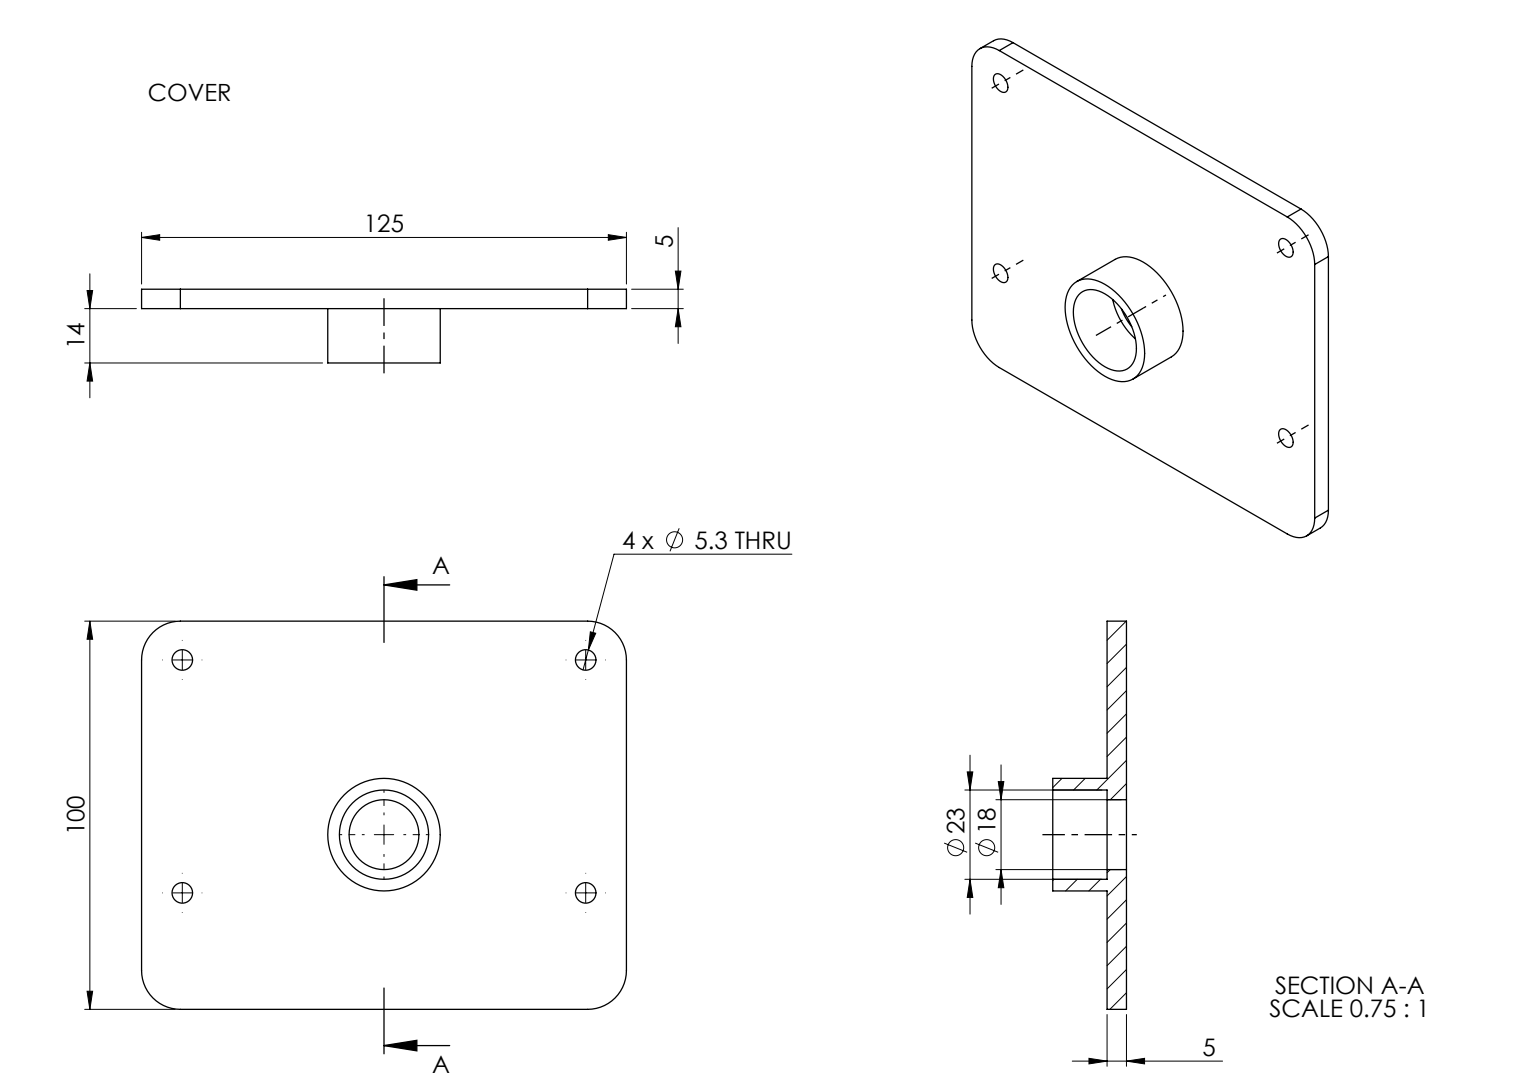
ISO-10303-21;
HEADER;
FILE_DESCRIPTION (('STEP AP214'),
    '1' );
FILE_NAME ('cover.step',
    '2026-10-03T12:29:21',
    ( '' ),
    ( '' ),
    'SwSTEP 2.0',
    'SolidWorks 2026',
    '' );
FILE_SCHEMA (( 'AUTOMOTIVE_DESIGN' ));
ENDSEC;

DATA;
#54=DIRECTION ( 'NONE',  ( 0.000000000000000000, -1.000000000000000000, 0.000000000000000000 ) ) ;
#65=VERTEX_POINT ( 'NONE', #16100 ) ;
#67=CARTESIAN_POINT ( 'NONE',  ( 0.000000000000000000, 0.000000000000000000, 0.000000000000000000 ) ) ;
#103=FILL_AREA_STYLE_COLOUR ( '', #1898 ) ;
#122=CARTESIAN_POINT ( 'NONE',  ( 0.000000000000000000, 0.000000000000000000, 5.000000000000000000 ) ) ;
#132=EDGE_CURVE ( 'NONE', #3302, #4120, #4083, .T. ) ;
#140=FACE_OUTER_BOUND ( 'NONE', #16746, .T. ) ;
#173=DIRECTION ( 'NONE',  ( 0.000000000000000000, 0.000000000000000000, 1.000000000000000000 ) ) ;
#185=DIRECTION ( 'NONE',  ( 1.000000000000000000, 0.000000000000000000, 0.000000000000000000 ) ) ;
#194=DIRECTION ( 'NONE',  ( 1.000000000000000000, 0.000000000000000000, 0.000000000000000000 ) ) ;
#206=( NAMED_UNIT ( * ) SI_UNIT ( $, .STERADIAN. ) SOLID_ANGLE_UNIT ( ) );
#216=LINE ( 'NONE', #11142, #13413 ) ;
#238=CARTESIAN_POINT ( 'NONE',  ( -52.49999999999999289, -30.00000000000000000, 0.000000000000000000 ) ) ;
#249=DIRECTION ( 'NONE',  ( -0.000000000000000000, -0.000000000000000000, 1.000000000000000000 ) ) ;
#257=LINE ( 'NONE', #14576, #12551 ) ;
#270=EDGE_LOOP ( 'NONE', ( #12954, #8026, #4477, #571 ) ) ;
#286=PRODUCT_CONTEXT ( 'NONE', #3554, 'mechanical' ) ;
#314=DIRECTION ( 'NONE',  ( -0.000000000000000000, -0.000000000000000000, 1.000000000000000000 ) ) ;
#324=ORIENTED_EDGE ( 'NONE', *, *, #1202, .T. ) ;
#327=ORIENTED_EDGE ( 'NONE', *, *, #8085, .T. ) ;
#333=DIRECTION ( 'NONE',  ( -1.000000000000000000, 0.000000000000000000, 0.000000000000000000 ) ) ;
#349=VERTEX_POINT ( 'NONE', #17246 ) ;
#368=EDGE_LOOP ( 'NONE', ( #9390, #15256, #3341, #1635, #4917, #19563, #12589, #1221 ) ) ;
#456=DIRECTION ( 'NONE',  ( -0.000000000000000000, -0.000000000000000000, 1.000000000000000000 ) ) ;
#457=AXIS2_PLACEMENT_3D ( 'NONE', #13399, #8610, #18470 ) ;
#459=DIRECTION ( 'NONE',  ( 1.000000000000000000, 0.000000000000000000, 0.000000000000000000 ) ) ;
#487=ORIENTED_EDGE ( 'NONE', *, *, #16093, .F. ) ;
#546=ADVANCED_FACE ( 'NONE', ( #140 ), #19233, .F. ) ;
#571=ORIENTED_EDGE ( 'NONE', *, *, #18719, .T. ) ;
#595=CIRCLE ( 'NONE', #8055, 14.49999999999999822 ) ;
#600=DIRECTION ( 'NONE',  ( 1.000000000000000000, 0.000000000000000000, 0.000000000000000000 ) ) ;
#613=CARTESIAN_POINT ( 'NONE',  ( -54.64999999999999858, -39.99999999999999289, 5.000000000000000000 ) ) ;
#618=DIRECTION ( 'NONE',  ( 0.000000000000000000, 0.000000000000000000, 1.000000000000000000 ) ) ;
#742=VERTEX_POINT ( 'NONE', #7013 ) ;
#768=ORIENTED_EDGE ( 'NONE', *, *, #3979, .F. ) ;
#778=EDGE_CURVE ( 'NONE', #4723, #14352, #12593, .T. ) ;
#848=ORIENTED_EDGE ( 'NONE', *, *, #778, .T. ) ;
#856=FACE_BOUND ( 'NONE', #9647, .T. ) ;
#880=VERTEX_POINT ( 'NONE', #4466 ) ;
#891=MECHANICAL_DESIGN_GEOMETRIC_PRESENTATION_REPRESENTATION('',(#4227),#19831);
#901=ORIENTED_EDGE ( 'NONE', *, *, #12581, .T. ) ;
#929=AXIS2_PLACEMENT_3D ( 'NONE', #67, #17673, #6521 ) ;
#960=DIRECTION ( 'NONE',  ( 0.000000000000000000, 0.000000000000000000, 1.000000000000000000 ) ) ;
#981=SURFACE_STYLE_USAGE ( .BOTH. , #14017 ) ;
#1001=CARTESIAN_POINT ( 'NONE',  ( -62.49999999999999289, -40.00000000000000000, 0.000000000000000000 ) ) ;
#1006=ORIENTED_EDGE ( 'NONE', *, *, #7889, .T. ) ;
#1032=DIRECTION ( 'NONE',  ( 0.000000000000000000, 0.000000000000000000, 1.000000000000000000 ) ) ;
#1035=CARTESIAN_POINT ( 'NONE',  ( 1.040949779275250179E-14, -85.00000000000000000, 19.00000000000000000 ) ) ;
#1057=CARTESIAN_POINT ( 'NONE',  ( 52.00000000000000000, -99.99999999999998579, 5.000000000000000000 ) ) ;
#1061=VERTEX_POINT ( 'NONE', #17520 ) ;
#1065=EDGE_LOOP ( 'NONE', ( #17257, #14549, #3120, #18251 ) ) ;
#1073=ORIENTED_EDGE ( 'NONE', *, *, #4313, .T. ) ;
#1110=CYLINDRICAL_SURFACE ( 'NONE', #14068, 10.00000000000000178 ) ;
#1168=CIRCLE ( 'NONE', #13352, 2.649999999999999467 ) ;
#1190=DIRECTION ( 'NONE',  ( -0.000000000000000000, -0.000000000000000000, 1.000000000000000000 ) ) ;
#1196=FILL_AREA_STYLE ('',( #10623 ) ) ;
#1202=EDGE_CURVE ( 'NONE', #20933, #12828, #18015, .T. ) ;
#1221=ORIENTED_EDGE ( 'NONE', *, *, #7003, .T. ) ;
#1227=VERTEX_POINT ( 'NONE', #3598 ) ;
#1239=DIRECTION ( 'NONE',  ( -0.000000000000000000, 0.000000000000000000, 1.000000000000000000 ) ) ;
#1264=ORIENTED_EDGE ( 'NONE', *, *, #19475, .F. ) ;
#1399=LINE ( 'NONE', #15489, #20347 ) ;
#1407=ORIENTED_EDGE ( 'NONE', *, *, #9613, .T. ) ;
#1414=FACE_BOUND ( 'NONE', #12896, .T. ) ;
#1419=CARTESIAN_POINT ( 'NONE',  ( -52.49999999999999289, -40.00000000000000000, 5.000000000000000000 ) ) ;
#1471=CIRCLE ( 'NONE', #19391, 8.999999999999998224 ) ;
#1510=EDGE_CURVE ( 'NONE', #880, #7974, #1471, .T. ) ;
#1511=LINE ( 'NONE', #14435, #17019 ) ;
#1525=ORIENTED_EDGE ( 'NONE', *, *, #2233, .F. ) ;
#1533=FACE_OUTER_BOUND ( 'NONE', #4714, .T. ) ;
#1548=CARTESIAN_POINT ( 'NONE',  ( 62.49999999999999289, -30.00000000000000000, 5.000000000000000000 ) ) ;
#1551=DIRECTION ( 'NONE',  ( 1.000000000000000000, 0.000000000000000000, 0.000000000000000000 ) ) ;
#1569=FACE_BOUND ( 'NONE', #6597, .T. ) ;
#1633=FACE_OUTER_BOUND ( 'NONE', #20105, .T. ) ;
#1635=ORIENTED_EDGE ( 'NONE', *, *, #6502, .T. ) ;
#1647=CARTESIAN_POINT ( 'NONE',  ( 9.000000000000007105, -85.00000000000000000, 5.000000000000000000 ) ) ;
#1650=ORIENTED_EDGE ( 'NONE', *, *, #1510, .F. ) ;
#1717=VERTEX_POINT ( 'NONE', #20608 ) ;
#1779=ORIENTED_EDGE ( 'NONE', *, *, #5333, .F. ) ;
#1803=SURFACE_STYLE_USAGE ( .BOTH. , #8258 ) ;
#1835=ORIENTED_EDGE ( 'NONE', *, *, #3908, .F. ) ;
#1844=DIRECTION ( 'NONE',  ( 1.000000000000000000, 0.000000000000000000, 0.000000000000000000 ) ) ;
#1855=CARTESIAN_POINT ( 'NONE',  ( 1.040949779275250179E-14, -85.00000000000000000, 5.000000000000000000 ) ) ;
#1898=COLOUR_RGB ( '', 0.66274510, 0.83137255, 0.94901961) ;
#1925=DIRECTION ( 'NONE',  ( -0.000000000000000000, -0.000000000000000000, -1.000000000000000000 ) ) ;
#1974=ADVANCED_FACE ( 'NONE', ( #11586 ), #11485, .F. ) ;
#1980=EDGE_LOOP ( 'NONE', ( #1407, #18308 ) ) ;
#1987=DIRECTION ( 'NONE',  ( 1.000000000000000000, 0.000000000000000000, 0.000000000000000000 ) ) ;
#1998=DIRECTION ( 'NONE',  ( 1.000000000000000000, 0.000000000000000000, -0.000000000000000000 ) ) ;
#2038=DIRECTION ( 'NONE',  ( -0.000000000000000000, 0.000000000000000000, 1.000000000000000000 ) ) ;
#2039=ORIENTED_EDGE ( 'NONE', *, *, #20622, .T. ) ;
#2116=VECTOR ( 'NONE', #12051, 1000.000000000000000 ) ;
#2147=EDGE_CURVE ( 'NONE', #10416, #11011, #18051, .T. ) ;
#2185=CARTESIAN_POINT ( 'NONE',  ( -52.00000000000000000, -39.99999999999999289, 5.000000000000000000 ) ) ;
#2226=EDGE_LOOP ( 'NONE', ( #10599, #3285, #1650, #3524 ) ) ;
#2228=DIRECTION ( 'NONE',  ( -0.000000000000000000, -0.000000000000000000, 1.000000000000000000 ) ) ;
#2229=ORIENTED_EDGE ( 'NONE', *, *, #14858, .F. ) ;
#2233=EDGE_CURVE ( 'NONE', #5012, #8902, #15023, .T. ) ;
#2270=AXIS2_PLACEMENT_3D ( 'NONE', #5785, #4208, #12376 ) ;
#2283=EDGE_LOOP ( 'NONE', ( #8472, #7507, #18183, #15740 ) ) ;
#2337=ORIENTED_EDGE ( 'NONE', *, *, #19059, .T. ) ;
#2376=EDGE_LOOP ( 'NONE', ( #8040, #13146, #1073, #324 ) ) ;
#2402=EDGE_LOOP ( 'NONE', ( #17842, #5849 ) ) ;
#2467=CARTESIAN_POINT ( 'NONE',  ( -11.49999999999998934, -85.00000000000000000, 19.00000000000000000 ) ) ;
#2481=CIRCLE ( 'NONE', #18048, 8.999999999999998224 ) ;
#2500=EDGE_LOOP ( 'NONE', ( #17069, #5268, #8184, #2039 ) ) ;
#2507=DIRECTION ( 'NONE',  ( 1.000000000000000000, 0.000000000000000000, 0.000000000000000000 ) ) ;
#2635=ORIENTED_EDGE ( 'NONE', *, *, #8017, .T. ) ;
#2645=CARTESIAN_POINT ( 'NONE',  ( -52.49999999999999289, -40.00000000000000000, 5.000000000000000000 ) ) ;
#2647=EDGE_CURVE ( 'NONE', #11011, #10416, #20768, .T. ) ;
#2665=ORIENTED_EDGE ( 'NONE', *, *, #5993, .F. ) ;
#2685=ADVANCED_FACE ( 'NONE', ( #16748 ), #5195, .F. ) ;
#2709=CARTESIAN_POINT ( 'NONE',  ( -49.35000000000000142, -99.99999999999998579, 0.000000000000000000 ) ) ;
#2717=CIRCLE ( 'NONE', #4068, 8.999999999999998224 ) ;
#2731=EDGE_CURVE ( 'NONE', #7766, #14029, #20375, .T. ) ;
#2755=ORIENTED_EDGE ( 'NONE', *, *, #6976, .T. ) ;
#2767=AXIS2_PLACEMENT_3D ( 'NONE', #12595, #19062, #7495 ) ;
#2803=ORIENTED_EDGE ( 'NONE', *, *, #8889, .T. ) ;
#2808=EDGE_LOOP ( 'NONE', ( #2337, #15718, #1779, #1264 ) ) ;
#2815=AXIS2_PLACEMENT_3D ( 'NONE', #1548, #5112, #17955 ) ;
#2970=VERTEX_POINT ( 'NONE', #6550 ) ;
#2988=CARTESIAN_POINT ( 'NONE',  ( -54.64999999999999858, -39.99999999999999289, 0.000000000000000000 ) ) ;
#2999=CARTESIAN_POINT ( 'NONE',  ( -62.49999999999999289, -130.0000000000000000, 5.000000000000000000 ) ) ;
#3022=ORIENTED_EDGE ( 'NONE', *, *, #6502, .F. ) ;
#3033=CARTESIAN_POINT ( 'NONE',  ( -62.49999999999999289, -30.00000000000000000, 5.000000000000000000 ) ) ;
#3036=SHAPE_REPRESENTATION ( 'cover', ( #12461 ), #5607 ) ;
#3088=DIRECTION ( 'NONE',  ( -0.000000000000000000, 0.000000000000000000, 1.000000000000000000 ) ) ;
#3120=ORIENTED_EDGE ( 'NONE', *, *, #19475, .T. ) ;
#3173=VECTOR ( 'NONE', #11996, 1000.000000000000000 ) ;
#3218=PLANE ( 'NONE',  #15694 ) ;
#3231=DIRECTION ( 'NONE',  ( 1.000000000000000000, 0.000000000000000000, 0.000000000000000000 ) ) ;
#3285=ORIENTED_EDGE ( 'NONE', *, *, #16985, .T. ) ;
#3293=DIRECTION ( 'NONE',  ( -0.000000000000000000, -0.000000000000000000, 1.000000000000000000 ) ) ;
#3302=VERTEX_POINT ( 'NONE', #11312 ) ;
#3313=AXIS2_PLACEMENT_3D ( 'NONE', #1035, #7484, #9299 ) ;
#3316=VECTOR ( 'NONE', #4614, 1000.000000000000000 ) ;
#3324=DIRECTION ( 'NONE',  ( 1.000000000000000000, 0.000000000000000000, -0.000000000000000000 ) ) ;
#3341=ORIENTED_EDGE ( 'NONE', *, *, #10133, .F. ) ;
#3361=DIRECTION ( 'NONE',  ( 0.000000000000000000, 0.000000000000000000, 1.000000000000000000 ) ) ;
#3401=ORIENTED_EDGE ( 'NONE', *, *, #2147, .T. ) ;
#3461=VECTOR ( 'NONE', #15119, 1000.000000000000000 ) ;
#3476=SHAPE_REPRESENTATION_RELATIONSHIP ( 'NONE' , 'NONE' ,  #3036, #7906 ) ;
#3483=EDGE_CURVE ( 'NONE', #5992, #9439, #11275, .T. ) ;
#3491=DIRECTION ( 'NONE',  ( 1.000000000000000000, 0.000000000000000000, 0.000000000000000000 ) ) ;
#3503=AXIS2_PLACEMENT_3D ( 'NONE', #3622, #456, #6905 ) ;
#3524=ORIENTED_EDGE ( 'NONE', *, *, #13526, .F. ) ;
#3528=CARTESIAN_POINT ( 'NONE',  ( -52.00000000000000000, -99.99999999999998579, 5.000000000000000000 ) ) ;
#3550=PRODUCT_DEFINITION_FORMATION_WITH_SPECIFIED_SOURCE ( 'ANY', '', #18644, .NOT_KNOWN. ) ;
#3554=APPLICATION_CONTEXT ( 'automotive_design' ) ;
#3585=DIRECTION ( 'NONE',  ( 1.000000000000000000, 0.000000000000000000, 0.000000000000000000 ) ) ;
#3594=DIRECTION ( 'NONE',  ( 1.000000000000000000, 0.000000000000000000, 0.000000000000000000 ) ) ;
#3598=CARTESIAN_POINT ( 'NONE',  ( 62.50000000000000000, -120.0000000000000142, 0.000000000000000000 ) ) ;
#3618=CIRCLE ( 'NONE', #11410, 11.50000000000000000 ) ;
#3622=CARTESIAN_POINT ( 'NONE',  ( 52.00000000000000000, -39.99999999999999289, 5.000000000000000000 ) ) ;
#3657=CYLINDRICAL_SURFACE ( 'NONE', #15141, 10.00000000000000178 ) ;
#3684=DIRECTION ( 'NONE',  ( -0.000000000000000000, -0.000000000000000000, -1.000000000000000000 ) ) ;
#3687=( NAMED_UNIT ( * ) PLANE_ANGLE_UNIT ( ) SI_UNIT ( $, .RADIAN. ) );
#3711=CARTESIAN_POINT ( 'NONE',  ( -52.00000000000000000, -99.99999999999998579, 5.000000000000000000 ) ) ;
#3728=LINE ( 'NONE', #4157, #20519 ) ;
#3748=DIRECTION ( 'NONE',  ( -1.000000000000000000, 0.000000000000000000, 0.000000000000000000 ) ) ;
#3874=LINE ( 'NONE', #613, #11834 ) ;
#3878=ORIENTED_EDGE ( 'NONE', *, *, #2731, .F. ) ;
#3880=PLANE ( 'NONE',  #9396 ) ;
#3889=FACE_OUTER_BOUND ( 'NONE', #11532, .T. ) ;
#3908=EDGE_CURVE ( 'NONE', #13107, #2970, #10106, .T. ) ;
#3979=EDGE_CURVE ( 'NONE', #9694, #4085, #257, .T. ) ;
#4002=DIRECTION ( 'NONE',  ( 1.000000000000000000, 0.000000000000000000, 0.000000000000000000 ) ) ;
#4016=FACE_BOUND ( 'NONE', #2402, .T. ) ;
#4023=PRODUCT_DEFINITION ( 'UNKNOWN', '', #3550, #5590 ) ;
#4051=CYLINDRICAL_SURFACE ( 'NONE', #16717, 14.49999999999999822 ) ;
#4068=AXIS2_PLACEMENT_3D ( 'NONE', #18351, #11993, #5102 ) ;
#4083=LINE ( 'NONE', #7161, #2116 ) ;
#4085=VERTEX_POINT ( 'NONE', #18364 ) ;
#4110=CYLINDRICAL_SURFACE ( 'NONE', #18878, 2.649999999999999467 ) ;
#4120=VERTEX_POINT ( 'NONE', #10204 ) ;
#4157=CARTESIAN_POINT ( 'NONE',  ( -8.999999999999987566, -85.00000000000000000, 5.000000000000000000 ) ) ;
#4208=DIRECTION ( 'NONE',  ( -0.000000000000000000, 0.000000000000000000, 1.000000000000000000 ) ) ;
#4227=STYLED_ITEM ( 'NONE', ( #5072 ), #7906 ) ;
#4257=AXIS2_PLACEMENT_3D ( 'NONE', #14702, #173, #16386 ) ;
#4273=DIRECTION ( 'NONE',  ( 0.000000000000000000, 0.000000000000000000, -1.000000000000000000 ) ) ;
#4277=FACE_OUTER_BOUND ( 'NONE', #7762, .T. ) ;
#4298=ADVANCED_FACE ( 'NONE', ( #1414, #1633 ), #16236, .T. ) ;
#4313=EDGE_CURVE ( 'NONE', #18213, #20933, #16332, .T. ) ;
#4338=DIRECTION ( 'NONE',  ( -0.000000000000000000, -0.000000000000000000, 1.000000000000000000 ) ) ;
#4344=ORIENTED_EDGE ( 'NONE', *, *, #132, .F. ) ;
#4405=ORIENTED_EDGE ( 'NONE', *, *, #13384, .T. ) ;
#4452=CARTESIAN_POINT ( 'NONE',  ( 49.35000000000000142, -39.99999999999999289, 5.000000000000000000 ) ) ;
#4466=CARTESIAN_POINT ( 'NONE',  ( -8.999999999999987566, -85.00000000000000000, 0.000000000000000000 ) ) ;
#4477=ORIENTED_EDGE ( 'NONE', *, *, #8889, .F. ) ;
#4501=DIRECTION ( 'NONE',  ( -0.000000000000000000, -0.000000000000000000, 1.000000000000000000 ) ) ;
#4545=DIRECTION ( 'NONE',  ( 1.000000000000000000, 0.000000000000000000, 0.000000000000000000 ) ) ;
#4576=DIRECTION ( 'NONE',  ( -0.000000000000000000, -0.000000000000000000, 1.000000000000000000 ) ) ;
#4585=CARTESIAN_POINT ( 'NONE',  ( -52.00000000000000000, -99.99999999999998579, 0.000000000000000000 ) ) ;
#4613=VECTOR ( 'NONE', #1190, 1000.000000000000000 ) ;
#4614=DIRECTION ( 'NONE',  ( -0.000000000000000000, -0.000000000000000000, 1.000000000000000000 ) ) ;
#4660=DIRECTION ( 'NONE',  ( 1.000000000000000000, 0.000000000000000000, 0.000000000000000000 ) ) ;
#4714=EDGE_LOOP ( 'NONE', ( #14546, #16819, #2635, #17037 ) ) ;
#4723=VERTEX_POINT ( 'NONE', #15893 ) ;
#4730=DIRECTION ( 'NONE',  ( 0.000000000000000000, 0.000000000000000000, 1.000000000000000000 ) ) ;
#4732=CIRCLE ( 'NONE', #16246, 14.49999999999999822 ) ;
#4757=VERTEX_POINT ( 'NONE', #16305 ) ;
#4781=CARTESIAN_POINT ( 'NONE',  ( 49.35000000000000142, -99.99999999999998579, 5.000000000000000000 ) ) ;
#4810=CIRCLE ( 'NONE', #2767, 2.649999999999999467 ) ;
#4838=FACE_OUTER_BOUND ( 'NONE', #368, .T. ) ;
#4897=DIRECTION ( 'NONE',  ( -0.000000000000000000, -0.000000000000000000, 1.000000000000000000 ) ) ;
#4901=DIRECTION ( 'NONE',  ( -0.000000000000000000, -0.000000000000000000, -1.000000000000000000 ) ) ;
#4917=ORIENTED_EDGE ( 'NONE', *, *, #9430, .F. ) ;
#5012=VERTEX_POINT ( 'NONE', #18627 ) ;
#5027=ORIENTED_EDGE ( 'NONE', *, *, #132, .T. ) ;
#5040=ORIENTED_EDGE ( 'NONE', *, *, #12921, .T. ) ;
#5072=PRESENTATION_STYLE_ASSIGNMENT (( #1803 ) ) ;
#5102=DIRECTION ( 'NONE',  ( 1.000000000000000000, 0.000000000000000000, 0.000000000000000000 ) ) ;
#5104=DIRECTION ( 'NONE',  ( -1.000000000000000000, -0.000000000000000000, -0.000000000000000000 ) ) ;
#5112=DIRECTION ( 'NONE',  ( -1.000000000000000000, -6.938893903907228378E-17, 0.000000000000000000 ) ) ;
#5113=EDGE_LOOP ( 'NONE', ( #5452, #8295, #1006, #18242 ) ) ;
#5174=DIRECTION ( 'NONE',  ( 0.000000000000000000, 0.000000000000000000, 1.000000000000000000 ) ) ;
#5175=CARTESIAN_POINT ( 'NONE',  ( 52.00000000000000000, -39.99999999999999289, 5.000000000000000000 ) ) ;
#5195=CYLINDRICAL_SURFACE ( 'NONE', #17686, 2.649999999999999467 ) ;
#5217=CARTESIAN_POINT ( 'NONE',  ( -49.35000000000000142, -99.99999999999998579, 5.000000000000000000 ) ) ;
#5267=AXIS2_PLACEMENT_3D ( 'NONE', #15050, #13251, #3594 ) ;
#5268=ORIENTED_EDGE ( 'NONE', *, *, #14560, .F. ) ;
#5293=CIRCLE ( 'NONE', #14825, 11.50000000000000000 ) ;
#5303=PLANE ( 'NONE',  #9025 ) ;
#5329=DIRECTION ( 'NONE',  ( 0.000000000000000000, -0.000000000000000000, 1.000000000000000000 ) ) ;
#5333=EDGE_CURVE ( 'NONE', #19867, #12993, #17798, .T. ) ;
#5340=EDGE_LOOP ( 'NONE', ( #9730, #6806 ) ) ;
#5425=DIRECTION ( 'NONE',  ( -0.000000000000000000, -0.000000000000000000, -1.000000000000000000 ) ) ;
#5432=VECTOR ( 'NONE', #5329, 1000.000000000000000 ) ;
#5446=CARTESIAN_POINT ( 'NONE',  ( 9.000000000000007105, -85.00000000000000000, 0.000000000000000000 ) ) ;
#5452=ORIENTED_EDGE ( 'NONE', *, *, #2647, .F. ) ;
#5538=DIRECTION ( 'NONE',  ( 1.000000000000000000, 0.000000000000000000, 0.000000000000000000 ) ) ;
#5584=CARTESIAN_POINT ( 'NONE',  ( 1.040949779275250179E-14, -85.00000000000000000, 5.000000000000000000 ) ) ;
#5590=PRODUCT_DEFINITION_CONTEXT ( 'detailed design', #18739, 'design' ) ;
#5606=CARTESIAN_POINT ( 'NONE',  ( -52.00000000000000000, -39.99999999999999289, 0.000000000000000000 ) ) ;
#5607=( GEOMETRIC_REPRESENTATION_CONTEXT ( 3 ) GLOBAL_UNCERTAINTY_ASSIGNED_CONTEXT ( ( #13245 ) ) GLOBAL_UNIT_ASSIGNED_CONTEXT ( ( #16006, #17399, #206 ) ) REPRESENTATION_CONTEXT ( 'NONE', 'WORKASPACE' ) );
#5642=ORIENTED_EDGE ( 'NONE', *, *, #12153, .F. ) ;
#5672=CARTESIAN_POINT ( 'NONE',  ( -62.49999999999999289, -40.00000000000000000, 5.000000000000000000 ) ) ;
#5701=DIRECTION ( 'NONE',  ( -0.000000000000000000, -0.000000000000000000, 1.000000000000000000 ) ) ;
#5710=ADVANCED_FACE ( 'NONE', ( #6894 ), #19721, .T. ) ;
#5768=VECTOR ( 'NONE', #4897, 1000.000000000000000 ) ;
#5770=EDGE_CURVE ( 'NONE', #65, #12993, #11564, .T. ) ;
#5785=CARTESIAN_POINT ( 'NONE',  ( 52.00000000000000000, -99.99999999999998579, 0.000000000000000000 ) ) ;
#5813=AXIS2_PLACEMENT_3D ( 'NONE', #15275, #2038, #459 ) ;
#5837=( LENGTH_UNIT ( ) NAMED_UNIT ( * ) SI_UNIT ( .MILLI., .METRE. ) );
#5849=ORIENTED_EDGE ( 'NONE', *, *, #17993, .F. ) ;
#5880=CARTESIAN_POINT ( 'NONE',  ( -14.49999999999998934, -85.00000000000000000, 19.00000000000000000 ) ) ;
#5899=DIRECTION ( 'NONE',  ( -0.000000000000000000, -0.000000000000000000, 1.000000000000000000 ) ) ;
#5957=CIRCLE ( 'NONE', #8653, 14.49999999999999822 ) ;
#5992=VERTEX_POINT ( 'NONE', #20461 ) ;
#5993=EDGE_CURVE ( 'NONE', #4723, #16392, #18982, .T. ) ;
#6071=ORIENTED_EDGE ( 'NONE', *, *, #2647, .T. ) ;
#6085=ORIENTED_EDGE ( 'NONE', *, *, #13384, .F. ) ;
#6109=ORIENTED_EDGE ( 'NONE', *, *, #7606, .F. ) ;
#6133=CYLINDRICAL_SURFACE ( 'NONE', #10043, 11.50000000000000000 ) ;
#6190=LINE ( 'NONE', #5880, #18085 ) ;
#6230=AXIS2_PLACEMENT_3D ( 'NONE', #3711, #13383, #15268 ) ;
#6300=CYLINDRICAL_SURFACE ( 'NONE', #7849, 10.00000000000000178 ) ;
#6308=ADVANCED_FACE ( 'NONE', ( #3889 ), #10370, .F. ) ;
#6329=CIRCLE ( 'NONE', #9721, 11.50000000000000000 ) ;
#6385=DIRECTION ( 'NONE',  ( -0.000000000000000000, -0.000000000000000000, 1.000000000000000000 ) ) ;
#6438=DIRECTION ( 'NONE',  ( 0.000000000000000000, 0.000000000000000000, 1.000000000000000000 ) ) ;
#6470=EDGE_LOOP ( 'NONE', ( #10872, #11075, #10292, #10874 ) ) ;
#6494=VECTOR ( 'NONE', #7893, 1000.000000000000000 ) ;
#6496=AXIS2_PLACEMENT_3D ( 'NONE', #13472, #6880, #18022 ) ;
#6502=EDGE_CURVE ( 'NONE', #1227, #15433, #17175, .T. ) ;
#6521=DIRECTION ( 'NONE',  ( 1.000000000000000000, 0.000000000000000000, 0.000000000000000000 ) ) ;
#6550=CARTESIAN_POINT ( 'NONE',  ( -62.49999999999999289, -120.0000000000000142, 5.000000000000000000 ) ) ;
#6555=ORIENTED_EDGE ( 'NONE', *, *, #10108, .T. ) ;
#6560=( NAMED_UNIT ( * ) SI_UNIT ( $, .STERADIAN. ) SOLID_ANGLE_UNIT ( ) );
#6562=DIRECTION ( 'NONE',  ( -6.938893903907228378E-17, 1.000000000000000000, -0.000000000000000000 ) ) ;
#6574=LINE ( 'NONE', #4781, #8598 ) ;
#6588=DIRECTION ( 'NONE',  ( -0.000000000000000000, -0.000000000000000000, -1.000000000000000000 ) ) ;
#6591=CARTESIAN_POINT ( 'NONE',  ( 1.040949779275250179E-14, -85.00000000000000000, 19.00000000000000000 ) ) ;
#6597=EDGE_LOOP ( 'NONE', ( #7651, #14778 ) ) ;
#6602=DIRECTION ( 'NONE',  ( -0.000000000000000000, -0.000000000000000000, 1.000000000000000000 ) ) ;
#6735=FACE_OUTER_BOUND ( 'NONE', #6470, .T. ) ;
#6794=DIRECTION ( 'NONE',  ( 1.000000000000000000, 0.000000000000000000, 0.000000000000000000 ) ) ;
#6806=ORIENTED_EDGE ( 'NONE', *, *, #11279, .T. ) ;
#6818=CIRCLE ( 'NONE', #16984, 10.00000000000000178 ) ;
#6880=DIRECTION ( 'NONE',  ( -0.000000000000000000, -0.000000000000000000, 1.000000000000000000 ) ) ;
#6890=FACE_BOUND ( 'NONE', #9412, .T. ) ;
#6894=FACE_OUTER_BOUND ( 'NONE', #15648, .T. ) ;
#6905=DIRECTION ( 'NONE',  ( 1.000000000000000000, 0.000000000000000000, 0.000000000000000000 ) ) ;
#6933=EDGE_LOOP ( 'NONE', ( #12931, #1835, #10041, #11228 ) ) ;
#6976=EDGE_CURVE ( 'NONE', #14029, #4120, #10974, .T. ) ;
#7003=EDGE_CURVE ( 'NONE', #10860, #9694, #19884, .T. ) ;
#7013=CARTESIAN_POINT ( 'NONE',  ( -14.49999999999998934, -85.00000000000000000, 5.000000000000000000 ) ) ;
#7072=DIRECTION ( 'NONE',  ( 0.000000000000000000, -0.000000000000000000, -1.000000000000000000 ) ) ;
#7161=CARTESIAN_POINT ( 'NONE',  ( 62.49999999999999289, -30.00000000000000000, 5.000000000000000000 ) ) ;
#7194=DIRECTION ( 'NONE',  ( -0.000000000000000000, 0.000000000000000000, 1.000000000000000000 ) ) ;
#7246=CARTESIAN_POINT ( 'NONE',  ( 14.50000000000000888, -85.00000000000000000, 19.00000000000000000 ) ) ;
#7309=FACE_OUTER_BOUND ( 'NONE', #10689, .T. ) ;
#7311=ORIENTED_EDGE ( 'NONE', *, *, #11837, .T. ) ;
#7326=ORIENTED_EDGE ( 'NONE', *, *, #3483, .T. ) ;
#7404=CARTESIAN_POINT ( 'NONE',  ( -52.49999999999999289, -120.0000000000000142, 0.000000000000000000 ) ) ;
#7445=DIRECTION ( 'NONE',  ( -0.000000000000000000, -0.000000000000000000, 1.000000000000000000 ) ) ;
#7449=ORIENTED_EDGE ( 'NONE', *, *, #778, .F. ) ;
#7484=DIRECTION ( 'NONE',  ( -0.000000000000000000, -0.000000000000000000, -1.000000000000000000 ) ) ;
#7495=DIRECTION ( 'NONE',  ( 1.000000000000000000, 0.000000000000000000, 0.000000000000000000 ) ) ;
#7507=ORIENTED_EDGE ( 'NONE', *, *, #12601, .T. ) ;
#7538=ORIENTED_EDGE ( 'NONE', *, *, #20247, .F. ) ;
#7548=PLANE ( 'NONE',  #13124 ) ;
#7574=AXIS2_PLACEMENT_3D ( 'NONE', #17587, #4338, #4545 ) ;
#7606=EDGE_CURVE ( 'NONE', #65, #13495, #5293, .T. ) ;
#7646=ORIENTED_EDGE ( 'NONE', *, *, #1510, .T. ) ;
#7651=ORIENTED_EDGE ( 'NONE', *, *, #12153, .T. ) ;
#7684=DIRECTION ( 'NONE',  ( -0.000000000000000000, -0.000000000000000000, -1.000000000000000000 ) ) ;
#7762=EDGE_LOOP ( 'NONE', ( #2665, #16982, #14718, #6555 ) ) ;
#7766=VERTEX_POINT ( 'NONE', #13552 ) ;
#7849=AXIS2_PLACEMENT_3D ( 'NONE', #12790, #8002, #14482 ) ;
#7871=EDGE_CURVE ( 'NONE', #4085, #4757, #6818, .T. ) ;
#7873=DIRECTION ( 'NONE',  ( 0.000000000000000000, 0.000000000000000000, -1.000000000000000000 ) ) ;
#7875=CARTESIAN_POINT ( 'NONE',  ( 52.00000000000000000, -39.99999999999999289, 5.000000000000000000 ) ) ;
#7884=ORIENTED_EDGE ( 'NONE', *, *, #18932, .T. ) ;
#7889=EDGE_CURVE ( 'NONE', #10195, #18098, #4810, .T. ) ;
#7892=ORIENTED_EDGE ( 'NONE', *, *, #11204, .F. ) ;
#7893=DIRECTION ( 'NONE',  ( -1.000000000000000000, -0.000000000000000000, -0.000000000000000000 ) ) ;
#7906=ADVANCED_BREP_SHAPE_REPRESENTATION ( '', ( #17220, #12461 ), #5607 ) ;
#7914=CIRCLE ( 'NONE', #14695, 2.649999999999999467 ) ;
#7918=DIRECTION ( 'NONE',  ( 1.000000000000000000, 0.000000000000000000, 0.000000000000000000 ) ) ;
#7949=AXIS2_PLACEMENT_3D ( 'NONE', #13257, #3088, #3491 ) ;
#7974=VERTEX_POINT ( 'NONE', #5446 ) ;
#7983=PLANE ( 'NONE',  #16662 ) ;
#7992=DIRECTION ( 'NONE',  ( 0.000000000000000000, 0.000000000000000000, 1.000000000000000000 ) ) ;
#8002=DIRECTION ( 'NONE',  ( -0.000000000000000000, 0.000000000000000000, -1.000000000000000000 ) ) ;
#8017=EDGE_CURVE ( 'NONE', #7766, #9694, #20400, .T. ) ;
#8022=CIRCLE ( 'NONE', #2270, 2.649999999999999467 ) ;
#8026=ORIENTED_EDGE ( 'NONE', *, *, #12068, .T. ) ;
#8040=ORIENTED_EDGE ( 'NONE', *, *, #12601, .F. ) ;
#8041=AXIS2_PLACEMENT_3D ( 'NONE', #8892, #16628, #15153 ) ;
#8055=AXIS2_PLACEMENT_3D ( 'NONE', #17271, #960, #4002 ) ;
#8067=DIRECTION ( 'NONE',  ( 1.000000000000000000, 0.000000000000000000, 0.000000000000000000 ) ) ;
#8079=DIRECTION ( 'NONE',  ( -0.000000000000000000, -0.000000000000000000, 1.000000000000000000 ) ) ;
#8085=EDGE_CURVE ( 'NONE', #14352, #4723, #20703, .T. ) ;
#8089=ADVANCED_FACE ( 'NONE', ( #20819 ), #6300, .T. ) ;
#8140=CARTESIAN_POINT ( 'NONE',  ( -11.49999999999998934, -85.00000000000000000, 5.000000000000000000 ) ) ;
#8163=AXIS2_PLACEMENT_3D ( 'NONE', #14475, #249, #9787 ) ;
#8184=ORIENTED_EDGE ( 'NONE', *, *, #11919, .T. ) ;
#8203=ADVANCED_FACE ( 'NONE', ( #1533 ), #7983, .F. ) ;
#8258=SURFACE_SIDE_STYLE ('',( #16415 ) ) ;
#8260=CYLINDRICAL_SURFACE ( 'NONE', #12236, 2.649999999999999467 ) ;
#8263=ADVANCED_FACE ( 'NONE', ( #20906 ), #13242, .F. ) ;
#8295=ORIENTED_EDGE ( 'NONE', *, *, #17680, .T. ) ;
#8325=DIRECTION ( 'NONE',  ( -0.000000000000000000, -0.000000000000000000, 1.000000000000000000 ) ) ;
#8364=( LENGTH_UNIT ( ) NAMED_UNIT ( * ) SI_UNIT ( .MILLI., .METRE. ) );
#8384=EDGE_LOOP ( 'NONE', ( #7892, #17588, #3878, #16103 ) ) ;
#8465=VERTEX_POINT ( 'NONE', #9103 ) ;
#8471=DIRECTION ( 'NONE',  ( 0.000000000000000000, -0.000000000000000000, -1.000000000000000000 ) ) ;
#8472=ORIENTED_EDGE ( 'NONE', *, *, #20095, .F. ) ;
#8493=DIRECTION ( 'NONE',  ( -0.000000000000000000, 0.000000000000000000, 1.000000000000000000 ) ) ;
#8533=DIRECTION ( 'NONE',  ( 1.000000000000000000, 0.000000000000000000, 0.000000000000000000 ) ) ;
#8568=UNCERTAINTY_MEASURE_WITH_UNIT (LENGTH_MEASURE( 1.000000000000000082E-05 ), #8364, 'distance_accuracy_value', 'NONE');
#8598=VECTOR ( 'NONE', #8079, 1000.000000000000000 ) ;
#8610=DIRECTION ( 'NONE',  ( -0.000000000000000000, 0.000000000000000000, 1.000000000000000000 ) ) ;
#8653=AXIS2_PLACEMENT_3D ( 'NONE', #18841, #1032, #17247 ) ;
#8696=ADVANCED_FACE ( 'NONE', ( #6735 ), #11510, .F. ) ;
#8864=FACE_OUTER_BOUND ( 'NONE', #5340, .T. ) ;
#8889=EDGE_CURVE ( 'NONE', #8465, #11004, #8964, .T. ) ;
#8892=CARTESIAN_POINT ( 'NONE',  ( -52.49999999999999289, -120.0000000000000142, 5.000000000000000000 ) ) ;
#8902=VERTEX_POINT ( 'NONE', #2709 ) ;
#8925=EDGE_CURVE ( 'NONE', #4757, #10860, #10673, .T. ) ;
#8941=LINE ( 'NONE', #18695, #10285 ) ;
#8964=LINE ( 'NONE', #17236, #10592 ) ;
#9003=CIRCLE ( 'NONE', #5267, 10.00000000000000178 ) ;
#9019=EDGE_LOOP ( 'NONE', ( #9158, #2755, #4344, #19574 ) ) ;
#9025=AXIS2_PLACEMENT_3D ( 'NONE', #13793, #20243, #18240 ) ;
#9053=CARTESIAN_POINT ( 'NONE',  ( 1.040949779275250179E-14, -85.00000000000000000, 19.00000000000000000 ) ) ;
#9073=ORIENTED_EDGE ( 'NONE', *, *, #20247, .T. ) ;
#9103=CARTESIAN_POINT ( 'NONE',  ( -52.49999999999999289, -130.0000000000000000, 5.000000000000000000 ) ) ;
#9112=DIRECTION ( 'NONE',  ( 0.000000000000000000, -0.000000000000000000, -1.000000000000000000 ) ) ;
#9158=ORIENTED_EDGE ( 'NONE', *, *, #10133, .T. ) ;
#9163=EDGE_CURVE ( 'NONE', #9439, #5992, #2481, .T. ) ;
#9190=COLOUR_RGB ( '', 0.66274510, 0.83137255, 0.94901961) ;
#9212=CARTESIAN_POINT ( 'NONE',  ( 1.040949779275250179E-14, -85.00000000000000000, 19.00000000000000000 ) ) ;
#9260=LINE ( 'NONE', #20688, #14383 ) ;
#9262=CYLINDRICAL_SURFACE ( 'NONE', #17408, 2.649999999999999467 ) ;
#9299=DIRECTION ( 'NONE',  ( -1.000000000000000000, 0.000000000000000000, 0.000000000000000000 ) ) ;
#9305=CARTESIAN_POINT ( 'NONE',  ( 52.50000000000000000, -120.0000000000000142, 0.000000000000000000 ) ) ;
#9390=ORIENTED_EDGE ( 'NONE', *, *, #8017, .F. ) ;
#9392=CIRCLE ( 'NONE', #8041, 10.00000000000000178 ) ;
#9396=AXIS2_PLACEMENT_3D ( 'NONE', #10360, #618, #1998 ) ;
#9400=AXIS2_PLACEMENT_3D ( 'NONE', #20822, #17960, #11392 ) ;
#9412=EDGE_LOOP ( 'NONE', ( #11224, #2229 ) ) ;
#9430=EDGE_CURVE ( 'NONE', #19301, #15433, #8941, .T. ) ;
#9439=VERTEX_POINT ( 'NONE', #15407 ) ;
#9458=DIRECTION ( 'NONE',  ( 0.000000000000000000, 1.000000000000000000, 0.000000000000000000 ) ) ;
#9468=ORIENTED_EDGE ( 'NONE', *, *, #3483, .F. ) ;
#9483=CARTESIAN_POINT ( 'NONE',  ( 52.00000000000000000, -39.99999999999999289, 0.000000000000000000 ) ) ;
#9486=ADVANCED_FACE ( 'NONE', ( #4277 ), #9262, .F. ) ;
#9566=DIRECTION ( 'NONE',  ( 0.000000000000000000, 0.000000000000000000, -1.000000000000000000 ) ) ;
#9613=EDGE_CURVE ( 'NONE', #18213, #349, #7914, .T. ) ;
#9634=DIRECTION ( 'NONE',  ( -0.000000000000000000, -0.000000000000000000, 1.000000000000000000 ) ) ;
#9647=EDGE_LOOP ( 'NONE', ( #6085, #16166 ) ) ;
#9662=DIRECTION ( 'NONE',  ( -0.000000000000000000, 0.000000000000000000, -1.000000000000000000 ) ) ;
#9694=VERTEX_POINT ( 'NONE', #238 ) ;
#9695=CARTESIAN_POINT ( 'NONE',  ( -62.49999999999999289, -120.0000000000000142, 5.000000000000000000 ) ) ;
#9721=AXIS2_PLACEMENT_3D ( 'NONE', #15994, #16299, #194 ) ;
#9730=ORIENTED_EDGE ( 'NONE', *, *, #14560, .T. ) ;
#9761=LINE ( 'NONE', #18018, #14398 ) ;
#9787=DIRECTION ( 'NONE',  ( 1.000000000000000000, 0.000000000000000000, 0.000000000000000000 ) ) ;
#9839=ORIENTED_EDGE ( 'NONE', *, *, #17993, .T. ) ;
#9845=FILL_AREA_STYLE ('',( #103 ) ) ;
#9875=EDGE_CURVE ( 'NONE', #1717, #18188, #19766, .T. ) ;
#9890=ORIENTED_EDGE ( 'NONE', *, *, #14826, .T. ) ;
#9953=CARTESIAN_POINT ( 'NONE',  ( -52.00000000000000000, -39.99999999999999289, 5.000000000000000000 ) ) ;
#9955=AXIS2_PLACEMENT_3D ( 'NONE', #19950, #7445, #13926 ) ;
#9969=VERTEX_POINT ( 'NONE', #20464 ) ;
#9984=EDGE_CURVE ( 'NONE', #3302, #1227, #1399, .T. ) ;
#10041=ORIENTED_EDGE ( 'NONE', *, *, #19081, .F. ) ;
#10043=AXIS2_PLACEMENT_3D ( 'NONE', #12292, #12615, #18767 ) ;
#10060=VECTOR ( 'NONE', #8325, 1000.000000000000000 ) ;
#10062=DIRECTION ( 'NONE',  ( 1.000000000000000000, 0.000000000000000000, 0.000000000000000000 ) ) ;
#10106=LINE ( 'NONE', #9695, #5432 ) ;
#10108=EDGE_CURVE ( 'NONE', #1061, #16392, #10546, .T. ) ;
#10113=ADVANCED_FACE ( 'NONE', ( #11350 ), #11541, .F. ) ;
#10133=EDGE_CURVE ( 'NONE', #1227, #14029, #1511, .T. ) ;
#10141=ADVANCED_FACE ( 'NONE', ( #17822 ), #8260, .F. ) ;
#10159=VECTOR ( 'NONE', #6588, 1000.000000000000000 ) ;
#10161=DIRECTION ( 'NONE',  ( 0.000000000000000000, -1.000000000000000000, 0.000000000000000000 ) ) ;
#10195=VERTEX_POINT ( 'NONE', #12074 ) ;
#10204=CARTESIAN_POINT ( 'NONE',  ( 62.49999999999999289, -40.00000000000000000, 5.000000000000000000 ) ) ;
#10275=EDGE_CURVE ( 'NONE', #4757, #2970, #18322, .T. ) ;
#10285=VECTOR ( 'NONE', #5538, 1000.000000000000000 ) ;
#10292=ORIENTED_EDGE ( 'NONE', *, *, #14776, .T. ) ;
#10360=CARTESIAN_POINT ( 'NONE',  ( 1.040949779275250179E-14, -85.00000000000000000, 19.00000000000000000 ) ) ;
#10370=CYLINDRICAL_SURFACE ( 'NONE', #17848, 8.999999999999998224 ) ;
#10416=VERTEX_POINT ( 'NONE', #16480 ) ;
#10421=CIRCLE ( 'NONE', #12451, 2.649999999999999467 ) ;
#10429=ORIENTED_EDGE ( 'NONE', *, *, #5993, .T. ) ;
#10444=ORIENTED_EDGE ( 'NONE', *, *, #8925, .T. ) ;
#10481=UNCERTAINTY_MEASURE_WITH_UNIT (LENGTH_MEASURE( 1.000000000000000082E-05 ), #5837, 'distance_accuracy_value', 'NONE');
#10497=FACE_BOUND ( 'NONE', #14926, .T. ) ;
#10546=CIRCLE ( 'NONE', #14946, 2.649999999999999467 ) ;
#10554=( GEOMETRIC_REPRESENTATION_CONTEXT ( 3 ) GLOBAL_UNCERTAINTY_ASSIGNED_CONTEXT ( ( #10481 ) ) GLOBAL_UNIT_ASSIGNED_CONTEXT ( ( #5837, #10732, #17197 ) ) REPRESENTATION_CONTEXT ( 'NONE', 'WORKASPACE' ) );
#10576=EDGE_LOOP ( 'NONE', ( #20411, #20444, #3022, #11146 ) ) ;
#10592=VECTOR ( 'NONE', #2507, 1000.000000000000000 ) ;
#10599=ORIENTED_EDGE ( 'NONE', *, *, #9163, .T. ) ;
#10623=FILL_AREA_STYLE_COLOUR ( '', #9190 ) ;
#10673=LINE ( 'NONE', #5672, #3461 ) ;
#10689=EDGE_LOOP ( 'NONE', ( #5027, #15214, #11790, #16228, #16214, #7884, #2803, #901 ) ) ;
#10732=( NAMED_UNIT ( * ) PLANE_ANGLE_UNIT ( ) SI_UNIT ( $, .RADIAN. ) );
#10774=ADVANCED_FACE ( 'NONE', ( #20798 ), #1110, .T. ) ;
#10788=ADVANCED_FACE ( 'NONE', ( #14039 ), #14241, .T. ) ;
#10860=VERTEX_POINT ( 'NONE', #1001 ) ;
#10872=ORIENTED_EDGE ( 'NONE', *, *, #17680, .F. ) ;
#10874=ORIENTED_EDGE ( 'NONE', *, *, #16093, .T. ) ;
#10921=EDGE_CURVE ( 'NONE', #14352, #1061, #15700, .T. ) ;
#10941=DIRECTION ( 'NONE',  ( 1.000000000000000000, 0.000000000000000000, 0.000000000000000000 ) ) ;
#10953=DIRECTION ( 'NONE',  ( 1.000000000000000000, 0.000000000000000000, 0.000000000000000000 ) ) ;
#10961=DIRECTION ( 'NONE',  ( 0.000000000000000000, 0.000000000000000000, 1.000000000000000000 ) ) ;
#10974=LINE ( 'NONE', #17016, #3316 ) ;
#11004=VERTEX_POINT ( 'NONE', #11037 ) ;
#11011=VERTEX_POINT ( 'NONE', #2988 ) ;
#11037=CARTESIAN_POINT ( 'NONE',  ( 52.50000000000000000, -130.0000000000000000, 5.000000000000000000 ) ) ;
#11059=CARTESIAN_POINT ( 'NONE',  ( 52.50000000000000000, -120.0000000000000142, 5.000000000000000000 ) ) ;
#11075=ORIENTED_EDGE ( 'NONE', *, *, #2147, .F. ) ;
#11092=ORIENTED_EDGE ( 'NONE', *, *, #11279, .F. ) ;
#11142=CARTESIAN_POINT ( 'NONE',  ( -62.49999999999999289, -30.00000000000000000, 0.000000000000000000 ) ) ;
#11146=ORIENTED_EDGE ( 'NONE', *, *, #9984, .F. ) ;
#11168=EDGE_CURVE ( 'NONE', #10860, #13107, #216, .T. ) ;
#11188=EDGE_LOOP ( 'NONE', ( #7449, #10429, #9890, #15166 ) ) ;
#11199=FACE_BOUND ( 'NONE', #1980, .T. ) ;
#11204=EDGE_CURVE ( 'NONE', #4120, #18964, #9003, .T. ) ;
#11224=ORIENTED_EDGE ( 'NONE', *, *, #1202, .F. ) ;
#11228=ORIENTED_EDGE ( 'NONE', *, *, #18719, .F. ) ;
#11236=CARTESIAN_POINT ( 'NONE',  ( 52.00000000000000000, -39.99999999999999289, 5.000000000000000000 ) ) ;
#11275=CIRCLE ( 'NONE', #16013, 8.999999999999998224 ) ;
#11279=EDGE_CURVE ( 'NONE', #9969, #16951, #5957, .T. ) ;
#11312=CARTESIAN_POINT ( 'NONE',  ( 62.50000000000000000, -120.0000000000000142, 5.000000000000000000 ) ) ;
#11322=VECTOR ( 'NONE', #5104, 1000.000000000000000 ) ;
#11350=FACE_OUTER_BOUND ( 'NONE', #2226, .T. ) ;
#11392=DIRECTION ( 'NONE',  ( 1.000000000000000000, 0.000000000000000000, 0.000000000000000000 ) ) ;
#11410=AXIS2_PLACEMENT_3D ( 'NONE', #9212, #4730, #19350 ) ;
#11485=PLANE ( 'NONE',  #2815 ) ;
#11510=CYLINDRICAL_SURFACE ( 'NONE', #19722, 2.649999999999999467 ) ;
#11532=EDGE_LOOP ( 'NONE', ( #16454, #7326, #13455, #19051 ) ) ;
#11541=CYLINDRICAL_SURFACE ( 'NONE', #19345, 8.999999999999998224 ) ;
#11562=MECHANICAL_DESIGN_GEOMETRIC_PRESENTATION_REPRESENTATION('',(#20343),#10554);
#11564=LINE ( 'NONE', #16437, #12409 ) ;
#11567=AXIS2_PLACEMENT_3D ( 'NONE', #9483, #1239, #1551 ) ;
#11576=FACE_OUTER_BOUND ( 'NONE', #13685, .T. ) ;
#11586=FACE_OUTER_BOUND ( 'NONE', #9019, .T. ) ;
#11619=SHAPE_DEFINITION_REPRESENTATION ( #18831, #3036 ) ;
#11646=DIRECTION ( 'NONE',  ( -0.000000000000000000, -0.000000000000000000, 1.000000000000000000 ) ) ;
#11664=DIRECTION ( 'NONE',  ( 1.000000000000000000, 0.000000000000000000, 0.000000000000000000 ) ) ;
#11790=ORIENTED_EDGE ( 'NONE', *, *, #18207, .T. ) ;
#11795=EDGE_LOOP ( 'NONE', ( #18501, #16067 ) ) ;
#11834=VECTOR ( 'NONE', #5899, 1000.000000000000000 ) ;
#11837=EDGE_CURVE ( 'NONE', #9969, #15420, #15419, .T. ) ;
#11840=FACE_BOUND ( 'NONE', #14194, .T. ) ;
#11919=EDGE_CURVE ( 'NONE', #16951, #742, #6190, .T. ) ;
#11993=DIRECTION ( 'NONE',  ( 0.000000000000000000, 0.000000000000000000, 1.000000000000000000 ) ) ;
#11996=DIRECTION ( 'NONE',  ( -0.000000000000000000, -0.000000000000000000, 1.000000000000000000 ) ) ;
#12011=VECTOR ( 'NONE', #54, 1000.000000000000000 ) ;
#12051=DIRECTION ( 'NONE',  ( -6.938893903907228378E-17, 1.000000000000000000, -0.000000000000000000 ) ) ;
#12068=EDGE_CURVE ( 'NONE', #15433, #11004, #15737, .T. ) ;
#12073=VECTOR ( 'NONE', #20177, 1000.000000000000000 ) ;
#12074=CARTESIAN_POINT ( 'NONE',  ( -54.64999999999999858, -39.99999999999999289, 5.000000000000000000 ) ) ;
#12094=AXIS2_PLACEMENT_3D ( 'NONE', #7404, #9112, #16075 ) ;
#12107=CARTESIAN_POINT ( 'NONE',  ( -49.35000000000000142, -39.99999999999999289, 5.000000000000000000 ) ) ;
#12153=EDGE_CURVE ( 'NONE', #8902, #5012, #1168, .T. ) ;
#12174=FACE_OUTER_BOUND ( 'NONE', #2376, .T. ) ;
#12217=FACE_OUTER_BOUND ( 'NONE', #8384, .T. ) ;
#12236=AXIS2_PLACEMENT_3D ( 'NONE', #9953, #3293, #13044 ) ;
#12274=DIRECTION ( 'NONE',  ( 1.000000000000000000, 0.000000000000000000, 0.000000000000000000 ) ) ;
#12292=CARTESIAN_POINT ( 'NONE',  ( 1.040949779275250179E-14, -85.00000000000000000, 19.00000000000000000 ) ) ;
#12376=DIRECTION ( 'NONE',  ( 1.000000000000000000, 0.000000000000000000, 0.000000000000000000 ) ) ;
#12409=VECTOR ( 'NONE', #1925, 1000.000000000000000 ) ;
#12451=AXIS2_PLACEMENT_3D ( 'NONE', #3528, #14984, #7918 ) ;
#12461=AXIS2_PLACEMENT_3D ( 'NONE', #19474, #3361, #185 ) ;
#12525=PRESENTATION_STYLE_ASSIGNMENT (( #981 ) ) ;
#12547=CARTESIAN_POINT ( 'NONE',  ( 52.00000000000000000, -99.99999999999998579, 0.000000000000000000 ) ) ;
#12551=VECTOR ( 'NONE', #6602, 1000.000000000000000 ) ;
#12581=EDGE_CURVE ( 'NONE', #11004, #3302, #12694, .T. ) ;
#12589=ORIENTED_EDGE ( 'NONE', *, *, #11168, .F. ) ;
#12593=CIRCLE ( 'NONE', #5813, 2.649999999999999467 ) ;
#12595=CARTESIAN_POINT ( 'NONE',  ( -52.00000000000000000, -39.99999999999999289, 5.000000000000000000 ) ) ;
#12601=EDGE_CURVE ( 'NONE', #349, #12828, #6574, .T. ) ;
#12602=FACE_OUTER_BOUND ( 'NONE', #2283, .T. ) ;
#12615=DIRECTION ( 'NONE',  ( -0.000000000000000000, -0.000000000000000000, -1.000000000000000000 ) ) ;
#12676=CIRCLE ( 'NONE', #3503, 2.649999999999999467 ) ;
#12694=CIRCLE ( 'NONE', #7949, 10.00000000000000178 ) ;
#12759=VECTOR ( 'NONE', #20701, 1000.000000000000000 ) ;
#12790=CARTESIAN_POINT ( 'NONE',  ( -52.49999999999999289, -120.0000000000000142, 5.000000000000000000 ) ) ;
#12828=VERTEX_POINT ( 'NONE', #15889 ) ;
#12837=ORIENTED_EDGE ( 'NONE', *, *, #8925, .F. ) ;
#12842=CARTESIAN_POINT ( 'NONE',  ( 1.040949779275250179E-14, -85.00000000000000000, 5.000000000000000000 ) ) ;
#12872=CARTESIAN_POINT ( 'NONE',  ( -14.49999999999998934, -85.00000000000000000, 19.00000000000000000 ) ) ;
#12896=EDGE_LOOP ( 'NONE', ( #13916, #9468 ) ) ;
#12904=LINE ( 'NONE', #14503, #10060 ) ;
#12921=EDGE_CURVE ( 'NONE', #12993, #19867, #6329, .T. ) ;
#12931=ORIENTED_EDGE ( 'NONE', *, *, #18932, .F. ) ;
#12954=ORIENTED_EDGE ( 'NONE', *, *, #9430, .T. ) ;
#12993=VERTEX_POINT ( 'NONE', #16404 ) ;
#13005=AXIS2_PLACEMENT_3D ( 'NONE', #4585, #19112, #10941 ) ;
#13044=DIRECTION ( 'NONE',  ( 1.000000000000000000, 0.000000000000000000, 0.000000000000000000 ) ) ;
#13075=ADVANCED_FACE ( 'NONE', ( #8864, #11840 ), #3880, .T. ) ;
#13107=VERTEX_POINT ( 'NONE', #19788 ) ;
#13120=DIRECTION ( 'NONE',  ( -0.000000000000000000, -0.000000000000000000, 1.000000000000000000 ) ) ;
#13124=AXIS2_PLACEMENT_3D ( 'NONE', #2999, #9458, #15919 ) ;
#13146=ORIENTED_EDGE ( 'NONE', *, *, #9613, .F. ) ;
#13163=DIRECTION ( 'NONE',  ( 1.000000000000000000, 0.000000000000000000, 0.000000000000000000 ) ) ;
#13242=CYLINDRICAL_SURFACE ( 'NONE', #15303, 2.649999999999999467 ) ;
#13245=UNCERTAINTY_MEASURE_WITH_UNIT (LENGTH_MEASURE( 1.000000000000000082E-05 ), #16006, 'distance_accuracy_value', 'NONE');
#13251=DIRECTION ( 'NONE',  ( -0.000000000000000000, 0.000000000000000000, 1.000000000000000000 ) ) ;
#13257=CARTESIAN_POINT ( 'NONE',  ( 52.50000000000000000, -120.0000000000000142, 5.000000000000000000 ) ) ;
#13259=ADVANCED_FACE ( 'NONE', ( #17355 ), #14188, .F. ) ;
#13284=CARTESIAN_POINT ( 'NONE',  ( -52.00000000000000000, -99.99999999999998579, 0.000000000000000000 ) ) ;
#13352=AXIS2_PLACEMENT_3D ( 'NONE', #13284, #8493, #1844 ) ;
#13383=DIRECTION ( 'NONE',  ( -0.000000000000000000, -0.000000000000000000, 1.000000000000000000 ) ) ;
#13384=EDGE_CURVE ( 'NONE', #18188, #1717, #10421, .T. ) ;
#13399=CARTESIAN_POINT ( 'NONE',  ( -52.00000000000000000, -39.99999999999999289, 0.000000000000000000 ) ) ;
#13413=VECTOR ( 'NONE', #17828, 1000.000000000000000 ) ;
#13455=ORIENTED_EDGE ( 'NONE', *, *, #13526, .T. ) ;
#13472=CARTESIAN_POINT ( 'NONE',  ( 52.00000000000000000, -99.99999999999998579, 5.000000000000000000 ) ) ;
#13495=VERTEX_POINT ( 'NONE', #2467 ) ;
#13526=EDGE_CURVE ( 'NONE', #9439, #880, #3728, .T. ) ;
#13550=DIRECTION ( 'NONE',  ( -1.000000000000000000, 0.000000000000000000, 0.000000000000000000 ) ) ;
#13552=CARTESIAN_POINT ( 'NONE',  ( 52.50000000000000000, -30.00000000000000000, 0.000000000000000000 ) ) ;
#13570=ORIENTED_EDGE ( 'NONE', *, *, #3908, .T. ) ;
#13668=DIRECTION ( 'NONE',  ( 1.000000000000000000, 0.000000000000000000, 0.000000000000000000 ) ) ;
#13685=EDGE_LOOP ( 'NONE', ( #17624, #13570, #19069, #10444 ) ) ;
#13699=ORIENTED_EDGE ( 'NONE', *, *, #15093, .T. ) ;
#13793=CARTESIAN_POINT ( 'NONE',  ( 0.000000000000000000, 0.000000000000000000, 5.000000000000000000 ) ) ;
#13881=CARTESIAN_POINT ( 'NONE',  ( 52.50000000000000000, -30.00000000000000000, 5.000000000000000000 ) ) ;
#13916=ORIENTED_EDGE ( 'NONE', *, *, #9163, .F. ) ;
#13926=DIRECTION ( 'NONE',  ( 1.000000000000000000, 0.000000000000000000, 0.000000000000000000 ) ) ;
#13997=EDGE_LOOP ( 'NONE', ( #19627, #5642, #9073, #4405 ) ) ;
#14013=ADVANCED_FACE ( 'NONE', ( #4016, #10497, #15375, #6890, #856, #7309 ), #5303, .T. ) ;
#14017=SURFACE_SIDE_STYLE ('',( #17083 ) ) ;
#14021=VECTOR ( 'NONE', #4501, 1000.000000000000000 ) ;
#14029=VERTEX_POINT ( 'NONE', #17601 ) ;
#14039=FACE_OUTER_BOUND ( 'NONE', #18139, .T. ) ;
#14068=AXIS2_PLACEMENT_3D ( 'NONE', #11059, #4273, #15924 ) ;
#14180=EDGE_LOOP ( 'NONE', ( #327, #848 ) ) ;
#14188=CYLINDRICAL_SURFACE ( 'NONE', #3313, 11.50000000000000000 ) ;
#14194=EDGE_LOOP ( 'NONE', ( #14823, #6109 ) ) ;
#14241=CYLINDRICAL_SURFACE ( 'NONE', #18123, 10.00000000000000178 ) ;
#14256=LINE ( 'NONE', #17554, #12759 ) ;
#14352=VERTEX_POINT ( 'NONE', #17889 ) ;
#14354=CIRCLE ( 'NONE', #16036, 14.49999999999999822 ) ;
#14359=AXIS2_PLACEMENT_3D ( 'NONE', #5606, #7194, #20015 ) ;
#14383=VECTOR ( 'NONE', #9566, 1000.000000000000000 ) ;
#14398=VECTOR ( 'NONE', #9662, 1000.000000000000000 ) ;
#14435=CARTESIAN_POINT ( 'NONE',  ( 62.49999999999999289, -30.00000000000000000, 0.000000000000000000 ) ) ;
#14455=FACE_OUTER_BOUND ( 'NONE', #270, .T. ) ;
#14461=CARTESIAN_POINT ( 'NONE',  ( -62.49999999999999289, -30.00000000000000000, 5.000000000000000000 ) ) ;
#14465=DIRECTION ( 'NONE',  ( -0.000000000000000000, 0.000000000000000000, 1.000000000000000000 ) ) ;
#14475=CARTESIAN_POINT ( 'NONE',  ( -52.00000000000000000, -99.99999999999998579, 5.000000000000000000 ) ) ;
#14482=DIRECTION ( 'NONE',  ( -1.000000000000000000, 0.000000000000000000, 0.000000000000000000 ) ) ;
#14503=CARTESIAN_POINT ( 'NONE',  ( -49.35000000000000142, -99.99999999999998579, 5.000000000000000000 ) ) ;
#14536=DIRECTION ( 'NONE',  ( -0.000000000000000000, -0.000000000000000000, -1.000000000000000000 ) ) ;
#14546=ORIENTED_EDGE ( 'NONE', *, *, #18207, .F. ) ;
#14549=ORIENTED_EDGE ( 'NONE', *, *, #7606, .T. ) ;
#14552=CARTESIAN_POINT ( 'NONE',  ( 54.64999999999999858, -99.99999999999998579, 5.000000000000000000 ) ) ;
#14560=EDGE_CURVE ( 'NONE', #16951, #9969, #14354, .T. ) ;
#14566=LINE ( 'NONE', #16349, #11322 ) ;
#14570=ADVANCED_FACE ( 'NONE', ( #11576 ), #3218, .F. ) ;
#14576=CARTESIAN_POINT ( 'NONE',  ( -52.49999999999999289, -30.00000000000000000, 5.000000000000000000 ) ) ;
#14695=AXIS2_PLACEMENT_3D ( 'NONE', #12547, #14465, #20909 ) ;
#14702=CARTESIAN_POINT ( 'NONE',  ( 1.040949779275250179E-14, -85.00000000000000000, 5.000000000000000000 ) ) ;
#14718=ORIENTED_EDGE ( 'NONE', *, *, #10921, .T. ) ;
#14776=EDGE_CURVE ( 'NONE', #10416, #18098, #18354, .T. ) ;
#14778=ORIENTED_EDGE ( 'NONE', *, *, #2233, .T. ) ;
#14803=FACE_BOUND ( 'NONE', #15890, .T. ) ;
#14823=ORIENTED_EDGE ( 'NONE', *, *, #19059, .F. ) ;
#14825=AXIS2_PLACEMENT_3D ( 'NONE', #19693, #5174, #10062 ) ;
#14826=EDGE_CURVE ( 'NONE', #16392, #1061, #12676, .T. ) ;
#14829=ORIENTED_EDGE ( 'NONE', *, *, #5333, .T. ) ;
#14858=EDGE_CURVE ( 'NONE', #12828, #20933, #18419, .T. ) ;
#14909=ADVANCED_FACE ( 'NONE', ( #15406 ), #4051, .T. ) ;
#14920=AXIS2_PLACEMENT_3D ( 'NONE', #122, #19302, #13163 ) ;
#14926=EDGE_LOOP ( 'NONE', ( #487, #17639 ) ) ;
#14931=ORIENTED_EDGE ( 'NONE', *, *, #7003, .F. ) ;
#14946=AXIS2_PLACEMENT_3D ( 'NONE', #11236, #314, #8067 ) ;
#14984=DIRECTION ( 'NONE',  ( -0.000000000000000000, -0.000000000000000000, 1.000000000000000000 ) ) ;
#15023=CIRCLE ( 'NONE', #13005, 2.649999999999999467 ) ;
#15050=CARTESIAN_POINT ( 'NONE',  ( 52.50000000000000000, -40.00000000000000000, 5.000000000000000000 ) ) ;
#15059=DIRECTION ( 'NONE',  ( 1.000000000000000000, 0.000000000000000000, 0.000000000000000000 ) ) ;
#15092=DIRECTION ( 'NONE',  ( -0.000000000000000000, -0.000000000000000000, -1.000000000000000000 ) ) ;
#15093=EDGE_CURVE ( 'NONE', #5012, #1717, #15827, .T. ) ;
#15111=CARTESIAN_POINT ( 'NONE',  ( 1.040949779275250179E-14, -85.00000000000000000, 5.000000000000000000 ) ) ;
#15119=DIRECTION ( 'NONE',  ( 0.000000000000000000, 0.000000000000000000, -1.000000000000000000 ) ) ;
#15141=AXIS2_PLACEMENT_3D ( 'NONE', #17209, #15602, #3748 ) ;
#15149=EDGE_CURVE ( 'NONE', #18964, #7766, #9260, .T. ) ;
#15153=DIRECTION ( 'NONE',  ( 1.000000000000000000, 0.000000000000000000, 0.000000000000000000 ) ) ;
#15166=ORIENTED_EDGE ( 'NONE', *, *, #10921, .F. ) ;
#15214=ORIENTED_EDGE ( 'NONE', *, *, #11204, .T. ) ;
#15256=ORIENTED_EDGE ( 'NONE', *, *, #2731, .T. ) ;
#15268=DIRECTION ( 'NONE',  ( 1.000000000000000000, 0.000000000000000000, 0.000000000000000000 ) ) ;
#15275=CARTESIAN_POINT ( 'NONE',  ( 52.00000000000000000, -39.99999999999999289, 0.000000000000000000 ) ) ;
#15303=AXIS2_PLACEMENT_3D ( 'NONE', #5175, #11646, #3585 ) ;
#15375=FACE_BOUND ( 'NONE', #11795, .T. ) ;
#15406=FACE_OUTER_BOUND ( 'NONE', #2500, .T. ) ;
#15407=CARTESIAN_POINT ( 'NONE',  ( -8.999999999999987566, -85.00000000000000000, 5.000000000000000000 ) ) ;
#15419=LINE ( 'NONE', #7246, #12073 ) ;
#15420=VERTEX_POINT ( 'NONE', #20249 ) ;
#15433=VERTEX_POINT ( 'NONE', #18567 ) ;
#15489=CARTESIAN_POINT ( 'NONE',  ( 62.50000000000000000, -120.0000000000000142, 5.000000000000000000 ) ) ;
#15553=DIRECTION ( 'NONE',  ( 1.000000000000000000, 0.000000000000000000, 0.000000000000000000 ) ) ;
#15590=CARTESIAN_POINT ( 'NONE',  ( 54.64999999999999858, -39.99999999999999289, 5.000000000000000000 ) ) ;
#15602=DIRECTION ( 'NONE',  ( 0.000000000000000000, 0.000000000000000000, -1.000000000000000000 ) ) ;
#15641=CARTESIAN_POINT ( 'NONE',  ( 49.35000000000000142, -39.99999999999999289, 5.000000000000000000 ) ) ;
#15648=EDGE_LOOP ( 'NONE', ( #11092, #7311, #9839, #16908 ) ) ;
#15694=AXIS2_PLACEMENT_3D ( 'NONE', #18050, #3324, #16350 ) ;
#15700=LINE ( 'NONE', #15590, #16120 ) ;
#15718=ORIENTED_EDGE ( 'NONE', *, *, #5770, .T. ) ;
#15737=LINE ( 'NONE', #19023, #14021 ) ;
#15740=ORIENTED_EDGE ( 'NONE', *, *, #4313, .F. ) ;
#15827=LINE ( 'NONE', #17315, #19117 ) ;
#15889=CARTESIAN_POINT ( 'NONE',  ( 49.35000000000000142, -99.99999999999998579, 5.000000000000000000 ) ) ;
#15890=EDGE_LOOP ( 'NONE', ( #3401, #6071 ) ) ;
#15893=CARTESIAN_POINT ( 'NONE',  ( 49.35000000000000142, -39.99999999999999289, 0.000000000000000000 ) ) ;
#15919=DIRECTION ( 'NONE',  ( 0.000000000000000000, -0.000000000000000000, 1.000000000000000000 ) ) ;
#15924=DIRECTION ( 'NONE',  ( -1.000000000000000000, 0.000000000000000000, 0.000000000000000000 ) ) ;
#15933=DIRECTION ( 'NONE',  ( 1.000000000000000000, 0.000000000000000000, 0.000000000000000000 ) ) ;
#15964=ADVANCED_FACE ( 'NONE', ( #12602 ), #19067, .F. ) ;
#15994=CARTESIAN_POINT ( 'NONE',  ( 1.040949779275250179E-14, -85.00000000000000000, 5.000000000000000000 ) ) ;
#16006=( LENGTH_UNIT ( ) NAMED_UNIT ( * ) SI_UNIT ( .MILLI., .METRE. ) );
#16013=AXIS2_PLACEMENT_3D ( 'NONE', #15111, #19970, #600 ) ;
#16036=AXIS2_PLACEMENT_3D ( 'NONE', #6591, #7992, #6794 ) ;
#16067=ORIENTED_EDGE ( 'NONE', *, *, #14826, .F. ) ;
#16075=DIRECTION ( 'NONE',  ( 1.000000000000000000, 0.000000000000000000, 0.000000000000000000 ) ) ;
#16093=EDGE_CURVE ( 'NONE', #18098, #10195, #18749, .T. ) ;
#16100=CARTESIAN_POINT ( 'NONE',  ( 11.50000000000001066, -85.00000000000000000, 19.00000000000000000 ) ) ;
#16103=ORIENTED_EDGE ( 'NONE', *, *, #15149, .F. ) ;
#16120=VECTOR ( 'NONE', #4576, 1000.000000000000000 ) ;
#16153=LINE ( 'NONE', #1647, #10159 ) ;
#16166=ORIENTED_EDGE ( 'NONE', *, *, #9875, .F. ) ;
#16168=CIRCLE ( 'NONE', #12094, 10.00000000000000178 ) ;
#16214=ORIENTED_EDGE ( 'NONE', *, *, #10275, .T. ) ;
#16228=ORIENTED_EDGE ( 'NONE', *, *, #7871, .T. ) ;
#16236=PLANE ( 'NONE',  #14920 ) ;
#16246=AXIS2_PLACEMENT_3D ( 'NONE', #20807, #10961, #15933 ) ;
#16249=CARTESIAN_POINT ( 'NONE',  ( 54.64999999999999858, -99.99999999999998579, 0.000000000000000000 ) ) ;
#16299=DIRECTION ( 'NONE',  ( 0.000000000000000000, 0.000000000000000000, 1.000000000000000000 ) ) ;
#16305=CARTESIAN_POINT ( 'NONE',  ( -62.49999999999999289, -40.00000000000000000, 5.000000000000000000 ) ) ;
#16321=AXIS2_PLACEMENT_3D ( 'NONE', #16537, #8471, #15059 ) ;
#16332=LINE ( 'NONE', #14552, #5768 ) ;
#16349=CARTESIAN_POINT ( 'NONE',  ( -62.49999999999999289, -30.00000000000000000, 5.000000000000000000 ) ) ;
#16350=DIRECTION ( 'NONE',  ( -0.000000000000000000, 0.000000000000000000, -1.000000000000000000 ) ) ;
#16384=PLANE ( 'NONE',  #929 ) ;
#16386=DIRECTION ( 'NONE',  ( 1.000000000000000000, 0.000000000000000000, 0.000000000000000000 ) ) ;
#16392=VERTEX_POINT ( 'NONE', #15641 ) ;
#16404=CARTESIAN_POINT ( 'NONE',  ( 11.50000000000001066, -85.00000000000000000, 5.000000000000000000 ) ) ;
#16415=SURFACE_STYLE_FILL_AREA ( #9845 ) ;
#16437=CARTESIAN_POINT ( 'NONE',  ( 11.50000000000001066, -85.00000000000000000, 19.00000000000000000 ) ) ;
#16454=ORIENTED_EDGE ( 'NONE', *, *, #16985, .F. ) ;
#16480=CARTESIAN_POINT ( 'NONE',  ( -49.35000000000000142, -39.99999999999999289, 0.000000000000000000 ) ) ;
#16508=CARTESIAN_POINT ( 'NONE',  ( -52.00000000000000000, -39.99999999999999289, 5.000000000000000000 ) ) ;
#16537=CARTESIAN_POINT ( 'NONE',  ( 52.50000000000000000, -40.00000000000000000, 0.000000000000000000 ) ) ;
#16595=CARTESIAN_POINT ( 'NONE',  ( 54.64999999999999858, -99.99999999999998579, 5.000000000000000000 ) ) ;
#16628=DIRECTION ( 'NONE',  ( -0.000000000000000000, 0.000000000000000000, 1.000000000000000000 ) ) ;
#16662=AXIS2_PLACEMENT_3D ( 'NONE', #14461, #10161, #7072 ) ;
#16687=CARTESIAN_POINT ( 'NONE',  ( -52.49999999999999289, -130.0000000000000000, 0.000000000000000000 ) ) ;
#16717=AXIS2_PLACEMENT_3D ( 'NONE', #9053, #15092, #16892 ) ;
#16746=EDGE_LOOP ( 'NONE', ( #1525, #13699, #16834, #7538 ) ) ;
#16748=FACE_OUTER_BOUND ( 'NONE', #13997, .T. ) ;
#16819=ORIENTED_EDGE ( 'NONE', *, *, #15149, .T. ) ;
#16834=ORIENTED_EDGE ( 'NONE', *, *, #9875, .T. ) ;
#16858=CARTESIAN_POINT ( 'NONE',  ( -52.00000000000000000, -99.99999999999998579, 5.000000000000000000 ) ) ;
#16892=DIRECTION ( 'NONE',  ( -1.000000000000000000, 0.000000000000000000, 0.000000000000000000 ) ) ;
#16908=ORIENTED_EDGE ( 'NONE', *, *, #11919, .F. ) ;
#16951=VERTEX_POINT ( 'NONE', #12872 ) ;
#16982=ORIENTED_EDGE ( 'NONE', *, *, #8085, .F. ) ;
#16984=AXIS2_PLACEMENT_3D ( 'NONE', #2645, #20542, #15553 ) ;
#16985=EDGE_CURVE ( 'NONE', #5992, #7974, #16153, .T. ) ;
#17016=CARTESIAN_POINT ( 'NONE',  ( 62.49999999999999289, -40.00000000000000000, 5.000000000000000000 ) ) ;
#17019=VECTOR ( 'NONE', #6562, 1000.000000000000000 ) ;
#17037=ORIENTED_EDGE ( 'NONE', *, *, #3979, .T. ) ;
#17069=ORIENTED_EDGE ( 'NONE', *, *, #11837, .F. ) ;
#17083=SURFACE_STYLE_FILL_AREA ( #1196 ) ;
#17120=EDGE_CURVE ( 'NONE', #7974, #880, #2717, .T. ) ;
#17175=CIRCLE ( 'NONE', #20884, 10.00000000000000178 ) ;
#17197=( NAMED_UNIT ( * ) SI_UNIT ( $, .STERADIAN. ) SOLID_ANGLE_UNIT ( ) );
#17209=CARTESIAN_POINT ( 'NONE',  ( 52.50000000000000000, -40.00000000000000000, 5.000000000000000000 ) ) ;
#17220=MANIFOLD_SOLID_BREP ( 'Extrude-Thin1', #17363 ) ;
#17236=CARTESIAN_POINT ( 'NONE',  ( -62.49999999999999289, -130.0000000000000000, 5.000000000000000000 ) ) ;
#17246=CARTESIAN_POINT ( 'NONE',  ( 49.35000000000000142, -99.99999999999998579, 0.000000000000000000 ) ) ;
#17247=DIRECTION ( 'NONE',  ( 1.000000000000000000, 0.000000000000000000, 0.000000000000000000 ) ) ;
#17257=ORIENTED_EDGE ( 'NONE', *, *, #5770, .F. ) ;
#17271=CARTESIAN_POINT ( 'NONE',  ( 1.040949779275250179E-14, -85.00000000000000000, 5.000000000000000000 ) ) ;
#17315=CARTESIAN_POINT ( 'NONE',  ( -54.64999999999999858, -99.99999999999998579, 5.000000000000000000 ) ) ;
#17355=FACE_OUTER_BOUND ( 'NONE', #1065, .T. ) ;
#17363=CLOSED_SHELL ( 'NONE', ( #19775, #5710, #10141, #8263, #15964, #546, #10113, #4298, #14013, #20274, #1974, #8203, #14570, #20575, #6308, #20381, #10774, #8089, #10788, #2685, #20646, #9486, #8696, #13075, #14909, #13259 ) ) ;
#17399=( NAMED_UNIT ( * ) PLANE_ANGLE_UNIT ( ) SI_UNIT ( $, .RADIAN. ) );
#17408=AXIS2_PLACEMENT_3D ( 'NONE', #7875, #20690, #10953 ) ;
#17520=CARTESIAN_POINT ( 'NONE',  ( 54.64999999999999858, -39.99999999999999289, 5.000000000000000000 ) ) ;
#17554=CARTESIAN_POINT ( 'NONE',  ( -11.49999999999998934, -85.00000000000000000, 19.00000000000000000 ) ) ;
#17582=DIRECTION ( 'NONE',  ( 0.000000000000000000, -0.000000000000000000, -1.000000000000000000 ) ) ;
#17587=CARTESIAN_POINT ( 'NONE',  ( 52.00000000000000000, -99.99999999999998579, 5.000000000000000000 ) ) ;
#17588=ORIENTED_EDGE ( 'NONE', *, *, #6976, .F. ) ;
#17601=CARTESIAN_POINT ( 'NONE',  ( 62.49999999999999289, -40.00000000000000000, 0.000000000000000000 ) ) ;
#17607=DIRECTION ( 'NONE',  ( 0.000000000000000000, 0.000000000000000000, -1.000000000000000000 ) ) ;
#17624=ORIENTED_EDGE ( 'NONE', *, *, #11168, .T. ) ;
#17639=ORIENTED_EDGE ( 'NONE', *, *, #7889, .F. ) ;
#17673=DIRECTION ( 'NONE',  ( -0.000000000000000000, 0.000000000000000000, 1.000000000000000000 ) ) ;
#17680=EDGE_CURVE ( 'NONE', #11011, #10195, #3874, .T. ) ;
#17686=AXIS2_PLACEMENT_3D ( 'NONE', #16858, #2228, #11664 ) ;
#17697=CARTESIAN_POINT ( 'NONE',  ( 1.040949779275250179E-14, -85.00000000000000000, 0.000000000000000000 ) ) ;
#17798=CIRCLE ( 'NONE', #4257, 11.50000000000000000 ) ;
#17822=FACE_OUTER_BOUND ( 'NONE', #5113, .T. ) ;
#17828=DIRECTION ( 'NONE',  ( 0.000000000000000000, -1.000000000000000000, 0.000000000000000000 ) ) ;
#17842=ORIENTED_EDGE ( 'NONE', *, *, #20622, .F. ) ;
#17848=AXIS2_PLACEMENT_3D ( 'NONE', #5584, #3684, #13550 ) ;
#17872=DIRECTION ( 'NONE',  ( 0.000000000000000000, 0.000000000000000000, 1.000000000000000000 ) ) ;
#17889=CARTESIAN_POINT ( 'NONE',  ( 54.64999999999999858, -39.99999999999999289, 0.000000000000000000 ) ) ;
#17955=DIRECTION ( 'NONE',  ( 6.938893903907228378E-17, -1.000000000000000000, 0.000000000000000000 ) ) ;
#17960=DIRECTION ( 'NONE',  ( 0.000000000000000000, -0.000000000000000000, -1.000000000000000000 ) ) ;
#17993=EDGE_CURVE ( 'NONE', #15420, #742, #4732, .T. ) ;
#18015=CIRCLE ( 'NONE', #6496, 2.649999999999999467 ) ;
#18018=CARTESIAN_POINT ( 'NONE',  ( -52.49999999999999289, -130.0000000000000000, 5.000000000000000000 ) ) ;
#18022=DIRECTION ( 'NONE',  ( 1.000000000000000000, 0.000000000000000000, 0.000000000000000000 ) ) ;
#18048=AXIS2_PLACEMENT_3D ( 'NONE', #1855, #17872, #3231 ) ;
#18050=CARTESIAN_POINT ( 'NONE',  ( -62.49999999999999289, -30.00000000000000000, 5.000000000000000000 ) ) ;
#18051=CIRCLE ( 'NONE', #457, 2.649999999999999467 ) ;
#18085=VECTOR ( 'NONE', #7684, 1000.000000000000000 ) ;
#18098=VERTEX_POINT ( 'NONE', #19130 ) ;
#18106=ORIENTED_EDGE ( 'NONE', *, *, #17120, .T. ) ;
#18123=AXIS2_PLACEMENT_3D ( 'NONE', #1419, #7873, #20487 ) ;
#18139=EDGE_LOOP ( 'NONE', ( #20789, #768, #14931, #12837 ) ) ;
#18146=AXIS2_PLACEMENT_3D ( 'NONE', #19826, #4901, #333 ) ;
#18183=ORIENTED_EDGE ( 'NONE', *, *, #14858, .T. ) ;
#18188=VERTEX_POINT ( 'NONE', #5217 ) ;
#18207=EDGE_CURVE ( 'NONE', #18964, #4085, #14566, .T. ) ;
#18213=VERTEX_POINT ( 'NONE', #16249 ) ;
#18240=DIRECTION ( 'NONE',  ( 1.000000000000000000, 0.000000000000000000, 0.000000000000000000 ) ) ;
#18242=ORIENTED_EDGE ( 'NONE', *, *, #14776, .F. ) ;
#18251=ORIENTED_EDGE ( 'NONE', *, *, #12921, .F. ) ;
#18308=ORIENTED_EDGE ( 'NONE', *, *, #20095, .T. ) ;
#18322=LINE ( 'NONE', #3033, #12011 ) ;
#18351=CARTESIAN_POINT ( 'NONE',  ( 1.040949779275250179E-14, -85.00000000000000000, 0.000000000000000000 ) ) ;
#18354=LINE ( 'NONE', #12107, #3173 ) ;
#18364=CARTESIAN_POINT ( 'NONE',  ( -52.49999999999999289, -30.00000000000000000, 5.000000000000000000 ) ) ;
#18419=CIRCLE ( 'NONE', #9955, 2.649999999999999467 ) ;
#18470=DIRECTION ( 'NONE',  ( 1.000000000000000000, 0.000000000000000000, 0.000000000000000000 ) ) ;
#18501=ORIENTED_EDGE ( 'NONE', *, *, #10108, .F. ) ;
#18567=CARTESIAN_POINT ( 'NONE',  ( 52.50000000000000000, -130.0000000000000000, 0.000000000000000000 ) ) ;
#18627=CARTESIAN_POINT ( 'NONE',  ( -54.64999999999999858, -99.99999999999998579, 0.000000000000000000 ) ) ;
#18644=PRODUCT ( 'cover', 'cover', '', ( #286 ) ) ;
#18695=CARTESIAN_POINT ( 'NONE',  ( -62.49999999999999289, -130.0000000000000000, 0.000000000000000000 ) ) ;
#18719=EDGE_CURVE ( 'NONE', #8465, #19301, #9761, .T. ) ;
#18739=APPLICATION_CONTEXT ( 'automotive_design' ) ;
#18749=CIRCLE ( 'NONE', #19099, 2.649999999999999467 ) ;
#18767=DIRECTION ( 'NONE',  ( -1.000000000000000000, 0.000000000000000000, 0.000000000000000000 ) ) ;
#18823=CARTESIAN_POINT ( 'NONE',  ( -62.49999999999999289, -30.00000000000000000, 0.000000000000000000 ) ) ;
#18831=PRODUCT_DEFINITION_SHAPE ( 'NONE', 'NONE',  #4023 ) ;
#18841=CARTESIAN_POINT ( 'NONE',  ( 1.040949779275250179E-14, -85.00000000000000000, 19.00000000000000000 ) ) ;
#18878=AXIS2_PLACEMENT_3D ( 'NONE', #1057, #5701, #13668 ) ;
#18932=EDGE_CURVE ( 'NONE', #2970, #8465, #9392, .T. ) ;
#18964=VERTEX_POINT ( 'NONE', #13881 ) ;
#18982=LINE ( 'NONE', #4452, #4613 ) ;
#19023=CARTESIAN_POINT ( 'NONE',  ( 52.50000000000000000, -130.0000000000000000, 5.000000000000000000 ) ) ;
#19051=ORIENTED_EDGE ( 'NONE', *, *, #17120, .F. ) ;
#19059=EDGE_CURVE ( 'NONE', #13495, #65, #3618, .T. ) ;
#19062=DIRECTION ( 'NONE',  ( -0.000000000000000000, -0.000000000000000000, 1.000000000000000000 ) ) ;
#19067=CYLINDRICAL_SURFACE ( 'NONE', #7574, 2.649999999999999467 ) ;
#19069=ORIENTED_EDGE ( 'NONE', *, *, #10275, .F. ) ;
#19081=EDGE_CURVE ( 'NONE', #19301, #13107, #16168, .T. ) ;
#19099=AXIS2_PLACEMENT_3D ( 'NONE', #16508, #9634, #1987 ) ;
#19112=DIRECTION ( 'NONE',  ( -0.000000000000000000, 0.000000000000000000, 1.000000000000000000 ) ) ;
#19117=VECTOR ( 'NONE', #6385, 1000.000000000000000 ) ;
#19130=CARTESIAN_POINT ( 'NONE',  ( -49.35000000000000142, -39.99999999999999289, 5.000000000000000000 ) ) ;
#19233=CYLINDRICAL_SURFACE ( 'NONE', #8163, 2.649999999999999467 ) ;
#19301=VERTEX_POINT ( 'NONE', #16687 ) ;
#19302=DIRECTION ( 'NONE',  ( -0.000000000000000000, 0.000000000000000000, 1.000000000000000000 ) ) ;
#19345=AXIS2_PLACEMENT_3D ( 'NONE', #12842, #14536, #19392 ) ;
#19350=DIRECTION ( 'NONE',  ( 1.000000000000000000, 0.000000000000000000, 0.000000000000000000 ) ) ;
#19353=FACE_BOUND ( 'NONE', #14180, .T. ) ;
#19391=AXIS2_PLACEMENT_3D ( 'NONE', #17697, #6438, #4660 ) ;
#19392=DIRECTION ( 'NONE',  ( -1.000000000000000000, 0.000000000000000000, 0.000000000000000000 ) ) ;
#19474=CARTESIAN_POINT ( 'NONE',  ( 0.000000000000000000, 0.000000000000000000, 0.000000000000000000 ) ) ;
#19475=EDGE_CURVE ( 'NONE', #13495, #19867, #14256, .T. ) ;
#19563=ORIENTED_EDGE ( 'NONE', *, *, #19081, .T. ) ;
#19564=FACE_BOUND ( 'NONE', #20165, .T. ) ;
#19574=ORIENTED_EDGE ( 'NONE', *, *, #9984, .T. ) ;
#19627=ORIENTED_EDGE ( 'NONE', *, *, #15093, .F. ) ;
#19693=CARTESIAN_POINT ( 'NONE',  ( 1.040949779275250179E-14, -85.00000000000000000, 19.00000000000000000 ) ) ;
#19721=CYLINDRICAL_SURFACE ( 'NONE', #18146, 14.49999999999999822 ) ;
#19722=AXIS2_PLACEMENT_3D ( 'NONE', #2185, #13120, #8533 ) ;
#19766=CIRCLE ( 'NONE', #6230, 2.649999999999999467 ) ;
#19775=ADVANCED_FACE ( 'NONE', ( #20651 ), #6133, .F. ) ;
#19788=CARTESIAN_POINT ( 'NONE',  ( -62.49999999999999289, -120.0000000000000142, 0.000000000000000000 ) ) ;
#19826=CARTESIAN_POINT ( 'NONE',  ( 1.040949779275250179E-14, -85.00000000000000000, 19.00000000000000000 ) ) ;
#19831=( GEOMETRIC_REPRESENTATION_CONTEXT ( 3 ) GLOBAL_UNCERTAINTY_ASSIGNED_CONTEXT ( ( #8568 ) ) GLOBAL_UNIT_ASSIGNED_CONTEXT ( ( #8364, #3687, #6560 ) ) REPRESENTATION_CONTEXT ( 'NONE', 'WORKASPACE' ) );
#19867=VERTEX_POINT ( 'NONE', #8140 ) ;
#19884=CIRCLE ( 'NONE', #9400, 10.00000000000000178 ) ;
#19950=CARTESIAN_POINT ( 'NONE',  ( 52.00000000000000000, -99.99999999999998579, 5.000000000000000000 ) ) ;
#19970=DIRECTION ( 'NONE',  ( 0.000000000000000000, 0.000000000000000000, 1.000000000000000000 ) ) ;
#20015=DIRECTION ( 'NONE',  ( 1.000000000000000000, 0.000000000000000000, 0.000000000000000000 ) ) ;
#20095=EDGE_CURVE ( 'NONE', #349, #18213, #8022, .T. ) ;
#20105=EDGE_LOOP ( 'NONE', ( #14829, #5040 ) ) ;
#20165=EDGE_LOOP ( 'NONE', ( #7646, #18106 ) ) ;
#20177=DIRECTION ( 'NONE',  ( -0.000000000000000000, -0.000000000000000000, -1.000000000000000000 ) ) ;
#20243=DIRECTION ( 'NONE',  ( -0.000000000000000000, 0.000000000000000000, 1.000000000000000000 ) ) ;
#20247=EDGE_CURVE ( 'NONE', #8902, #18188, #12904, .T. ) ;
#20249=CARTESIAN_POINT ( 'NONE',  ( 14.50000000000000888, -85.00000000000000000, 5.000000000000000000 ) ) ;
#20274=ADVANCED_FACE ( 'NONE', ( #14803, #19353, #11199, #1569, #4838, #19564 ), #16384, .F. ) ;
#20343=STYLED_ITEM ( 'NONE', ( #12525 ), #17220 ) ;
#20347=VECTOR ( 'NONE', #17607, 1000.000000000000000 ) ;
#20375=CIRCLE ( 'NONE', #16321, 10.00000000000000178 ) ;
#20381=ADVANCED_FACE ( 'NONE', ( #12217 ), #3657, .T. ) ;
#20400=LINE ( 'NONE', #18823, #6494 ) ;
#20411=ORIENTED_EDGE ( 'NONE', *, *, #12581, .F. ) ;
#20444=ORIENTED_EDGE ( 'NONE', *, *, #12068, .F. ) ;
#20461=CARTESIAN_POINT ( 'NONE',  ( 9.000000000000007105, -85.00000000000000000, 5.000000000000000000 ) ) ;
#20464=CARTESIAN_POINT ( 'NONE',  ( 14.50000000000000888, -85.00000000000000000, 19.00000000000000000 ) ) ;
#20487=DIRECTION ( 'NONE',  ( -1.000000000000000000, 0.000000000000000000, 0.000000000000000000 ) ) ;
#20519=VECTOR ( 'NONE', #5425, 1000.000000000000000 ) ;
#20542=DIRECTION ( 'NONE',  ( -0.000000000000000000, 0.000000000000000000, 1.000000000000000000 ) ) ;
#20575=ADVANCED_FACE ( 'NONE', ( #14455 ), #7548, .F. ) ;
#20608=CARTESIAN_POINT ( 'NONE',  ( -54.64999999999999858, -99.99999999999998579, 5.000000000000000000 ) ) ;
#20622=EDGE_CURVE ( 'NONE', #742, #15420, #595, .T. ) ;
#20646=ADVANCED_FACE ( 'NONE', ( #12174 ), #4110, .F. ) ;
#20651=FACE_OUTER_BOUND ( 'NONE', #2808, .T. ) ;
#20688=CARTESIAN_POINT ( 'NONE',  ( 52.50000000000000000, -30.00000000000000000, 5.000000000000000000 ) ) ;
#20690=DIRECTION ( 'NONE',  ( -0.000000000000000000, -0.000000000000000000, 1.000000000000000000 ) ) ;
#20701=DIRECTION ( 'NONE',  ( -0.000000000000000000, -0.000000000000000000, -1.000000000000000000 ) ) ;
#20703=CIRCLE ( 'NONE', #11567, 2.649999999999999467 ) ;
#20768=CIRCLE ( 'NONE', #14359, 2.649999999999999467 ) ;
#20789=ORIENTED_EDGE ( 'NONE', *, *, #7871, .F. ) ;
#20798=FACE_OUTER_BOUND ( 'NONE', #10576, .T. ) ;
#20807=CARTESIAN_POINT ( 'NONE',  ( 1.040949779275250179E-14, -85.00000000000000000, 5.000000000000000000 ) ) ;
#20819=FACE_OUTER_BOUND ( 'NONE', #6933, .T. ) ;
#20822=CARTESIAN_POINT ( 'NONE',  ( -52.49999999999999289, -40.00000000000000000, 0.000000000000000000 ) ) ;
#20884=AXIS2_PLACEMENT_3D ( 'NONE', #9305, #17582, #12274 ) ;
#20906=FACE_OUTER_BOUND ( 'NONE', #11188, .T. ) ;
#20909=DIRECTION ( 'NONE',  ( 1.000000000000000000, 0.000000000000000000, 0.000000000000000000 ) ) ;
#20933=VERTEX_POINT ( 'NONE', #16595 ) ;
ENDSEC;
END-ISO-10303-21;
